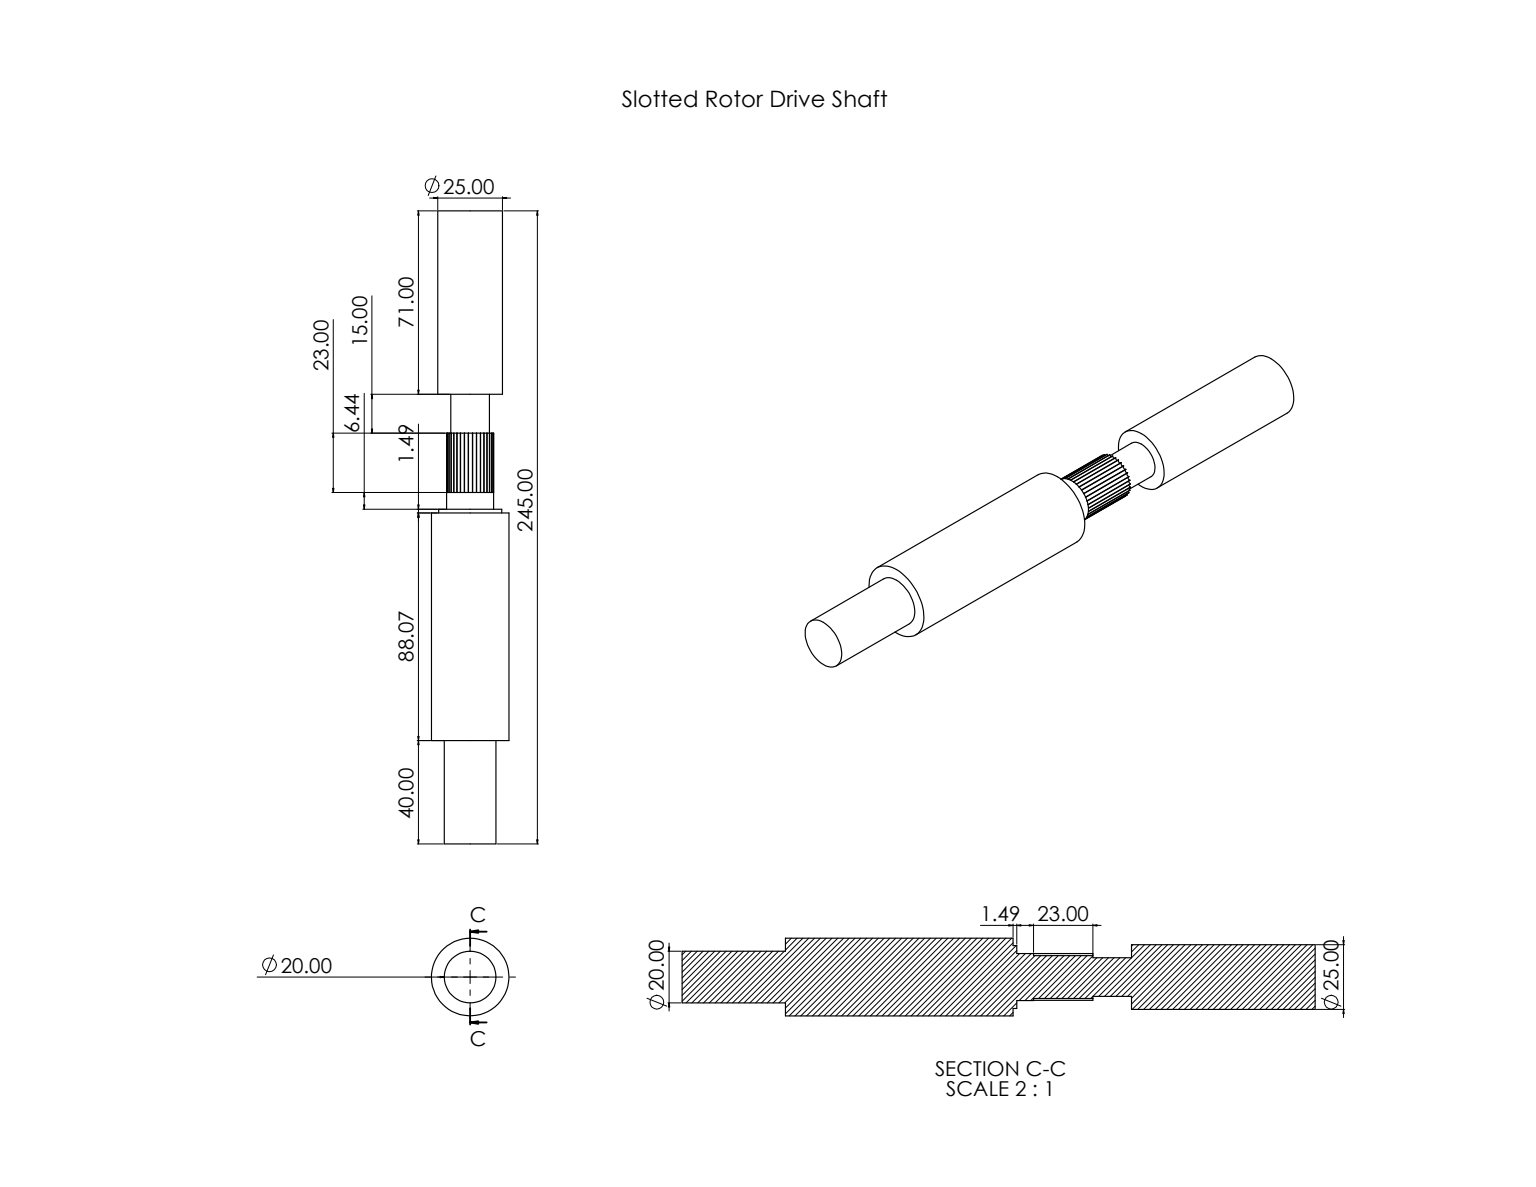
ISO-10303-21;
HEADER;
FILE_DESCRIPTION (('STEP AP214'),
    '1' );
FILE_NAME ('Slotted Rotor Drive Shaft.step',
    '2026-10-18T20:16:25',
    ( '' ),
    ( '' ),
    'SwSTEP 2.0',
    'SolidWorks 2025',
    '' );
FILE_SCHEMA (( 'AUTOMOTIVE_DESIGN' ));
ENDSEC;

DATA;
#10=DIRECTION ( 'NONE',  ( 1.000000000000000000, 0.000000000000000000, 0.000000000000000000 ) ) ;
#12=DIRECTION ( 'NONE',  ( 1.000000000000000000, 0.000000000000000000, 0.000000000000000000 ) ) ;
#34=VERTEX_POINT ( 'NONE', #489 ) ;
#36=DIRECTION ( 'NONE',  ( -0.000000000000000000, -0.000000000000000000, 1.000000000000000000 ) ) ;
#44=LINE ( 'NONE', #17187, #10483 ) ;
#51=CARTESIAN_POINT ( 'NONE',  ( 6.812559277181973627, -5.881244434206257310, 21.50000000000000000 ) ) ;
#57=DIRECTION ( 'NONE',  ( -0.000000000000000000, -0.000000000000000000, 1.000000000000000000 ) ) ;
#88=DIRECTION ( 'NONE',  ( 1.000000000000000000, 0.000000000000000000, 0.000000000000000000 ) ) ;
#89=ORIENTED_EDGE ( 'NONE', *, *, #20188, .F. ) ;
#101=CARTESIAN_POINT ( 'NONE',  ( 0.000000000000000000, 0.000000000000000000, -87.50000000000000000 ) ) ;
#103=ORIENTED_EDGE ( 'NONE', *, *, #23860, .T. ) ;
#107=CYLINDRICAL_SURFACE ( 'NONE', #23715, 10.00000000000003375 ) ;
#120=FACE_OUTER_BOUND ( 'NONE', #29698, .T. ) ;
#128=CARTESIAN_POINT ( 'NONE',  ( 0.000000000000000000, -2.435693370351110282E-15, 21.50000000000000355 ) ) ;
#141=ORIENTED_EDGE ( 'NONE', *, *, #9150, .T. ) ;
#157=ORIENTED_EDGE ( 'NONE', *, *, #6998, .F. ) ;
#163=DIRECTION ( 'NONE',  ( 1.000000000000000000, 0.000000000000000000, -0.000000000000000000 ) ) ;
#167=DIRECTION ( 'NONE',  ( 1.000000000000000000, 0.000000000000000000, 0.000000000000000000 ) ) ;
#168=LINE ( 'NONE', #19198, #17487 ) ;
#181=CARTESIAN_POINT ( 'NONE',  ( 3.993622308618880901, 8.159193615868410632, 21.50000000000000000 ) ) ;
#191=VERTEX_POINT ( 'NONE', #3449 ) ;
#193=CARTESIAN_POINT ( 'NONE',  ( 7.392982946727082449, -5.278755796068694828, -1.500000000000002442 ) ) ;
#222=DIRECTION ( 'NONE',  ( 0.000000000000000000, -1.132880637372608986E-16, 1.000000000000000000 ) ) ;
#233=DIRECTION ( 'NONE',  ( -0.000000000000000000, -0.000000000000000000, 1.000000000000000000 ) ) ;
#246=CARTESIAN_POINT ( 'NONE',  ( -7.856594496258223259, -4.390207617113929039, -1.500000000000002220 ) ) ;
#259=CARTESIAN_POINT ( 'NONE',  ( -8.268028093133393597, -3.763133143576407047, 13.22130136205108819 ) ) ;
#260=DIRECTION ( 'NONE',  ( -0.000000000000000000, 1.132880637372608986E-16, -1.000000000000000000 ) ) ;
#264=ORIENTED_EDGE ( 'NONE', *, *, #13066, .T. ) ;
#275=CIRCLE ( 'NONE', #26685, 10.00000000000003197 ) ;
#280=LINE ( 'NONE', #9800, #11506 ) ;
#299=ORIENTED_EDGE ( 'NONE', *, *, #13066, .F. ) ;
#352=EDGE_LOOP ( 'NONE', ( #24327, #26757, #11753, #27954 ) ) ;
#355=ORIENTED_EDGE ( 'NONE', *, *, #15805, .F. ) ;
#356=CIRCLE ( 'NONE', #4344, 0.7500000000000006661 ) ;
#371=AXIS2_PLACEMENT_3D ( 'NONE', #8358, #11002, #3982 ) ;
#376=EDGE_CURVE ( 'NONE', #10212, #10205, #7649, .T. ) ;
#384=VECTOR ( 'NONE', #1530, 1000.000000000000000 ) ;
#385=EDGE_LOOP ( 'NONE', ( #18527, #8717, #10000, #7620 ) ) ;
#386=VERTEX_POINT ( 'NONE', #5599 ) ;
#394=DIRECTION ( 'NONE',  ( 1.000000000000000000, 0.000000000000000000, -0.000000000000000000 ) ) ;
#396=CYLINDRICAL_SURFACE ( 'NONE', #20666, 0.7500000000000006661 ) ;
#398=ORIENTED_EDGE ( 'NONE', *, *, #13211, .T. ) ;
#411=DIRECTION ( 'NONE',  ( 1.000000000000000000, 0.000000000000000000, 0.000000000000000000 ) ) ;
#419=CARTESIAN_POINT ( 'NONE',  ( -0.6237340761795794331, 8.999114229549594057, -3.621320343559650379 ) ) ;
#426=CIRCLE ( 'NONE', #4407, 0.7500000000000006661 ) ;
#430=CARTESIAN_POINT ( 'NONE',  ( -5.881244434206279514, -6.812559277181949646, -3.621320343559650379 ) ) ;
#449=ADVANCED_FACE ( 'NONE', ( #17752 ), #28148, .F. ) ;
#454=VECTOR ( 'NONE', #3159, 1000.000000000000000 ) ;
#465=DIRECTION ( 'NONE',  ( 0.000000000000000000, -1.132880637372608986E-16, 1.000000000000000000 ) ) ;
#469=CARTESIAN_POINT ( 'NONE',  ( 8.752572334588121450, -2.431858781452763019, 13.22130136205108819 ) ) ;
#472=CARTESIAN_POINT ( 'NONE',  ( 7.856594496258195726, 4.390207617113981442, -3.621320343559650379 ) ) ;
#473=ORIENTED_EDGE ( 'NONE', *, *, #21967, .F. ) ;
#475=PLANE ( 'NONE',  #11721 ) ;
#478=DIRECTION ( 'NONE',  ( 0.000000000000000000, 0.000000000000000000, 1.000000000000000000 ) ) ;
#488=CARTESIAN_POINT ( 'NONE',  ( -2.431858781452794993, -8.752572334588114344, 13.22130136205108641 ) ) ;
#489=CARTESIAN_POINT ( 'NONE',  ( -7.749586724479453181, -2.959227181723774525, 21.50000000000000000 ) ) ;
#495=CIRCLE ( 'NONE', #13480, 0.7500000000000006661 ) ;
#504=CARTESIAN_POINT ( 'NONE',  ( 3.196529495465388226, 8.413215745755008967, 21.50000000000000000 ) ) ;
#507=ORIENTED_EDGE ( 'NONE', *, *, #26727, .T. ) ;
#513=EDGE_LOOP ( 'NONE', ( #8393, #2746, #22053, #19738 ) ) ;
#520=CARTESIAN_POINT ( 'NONE',  ( 3.993622308618881789, 8.159193615868410632, 13.22130136205108997 ) ) ;
#525=DIRECTION ( 'NONE',  ( -0.000000000000000000, -0.000000000000000000, 1.000000000000000000 ) ) ;
#533=PLANE ( 'NONE',  #14075 ) ;
#543=CARTESIAN_POINT ( 'NONE',  ( -3.914781618004754105, -8.197313248159934673, 13.22130136205108641 ) ) ;
#545=CARTESIAN_POINT ( 'NONE',  ( 5.278755796068665518, 7.392982946727100213, 13.22130136205108819 ) ) ;
#549=VERTEX_POINT ( 'NONE', #2245 ) ;
#556=ORIENTED_EDGE ( 'NONE', *, *, #19301, .T. ) ;
#557=DIRECTION ( 'NONE',  ( 0.000000000000000000, -1.132880637372608986E-16, 1.000000000000000000 ) ) ;
#564=DIRECTION ( 'NONE',  ( -0.000000000000000000, 1.132880637372608986E-16, -1.000000000000000000 ) ) ;
#583=DIRECTION ( 'NONE',  ( -0.000000000000000000, -0.000000000000000000, 1.000000000000000000 ) ) ;
#594=CIRCLE ( 'NONE', #15544, 9.084132297865673777 ) ;
#600=PLANE ( 'NONE',  #26319 ) ;
#604=CARTESIAN_POINT ( 'NONE',  ( 0.000000000000000000, -1.324687536737320328E-14, 29.43090101791767665 ) ) ;
#608=CARTESIAN_POINT ( 'NONE',  ( 0.000000000000000000, -2.435693370351110282E-15, 21.50000000000000355 ) ) ;
#610=AXIS2_PLACEMENT_3D ( 'NONE', #14293, #4786, #30528 ) ;
#620=EDGE_CURVE ( 'NONE', #21542, #7918, #19871, .T. ) ;
#630=VECTOR ( 'NONE', #11453, 1000.000000000000000 ) ;
#642=ORIENTED_EDGE ( 'NONE', *, *, #3488, .T. ) ;
#650=CARTESIAN_POINT ( 'NONE',  ( 0.000000000000000000, 12.49999999999999289, -16.50000000000000000 ) ) ;
#651=CARTESIAN_POINT ( 'NONE',  ( 8.499586724479435418, 2.959227181723830036, 21.50000000000000000 ) ) ;
#657=LINE ( 'NONE', #10172, #27987 ) ;
#662=LINE ( 'NONE', #10032, #18671 ) ;
#677=DIRECTION ( 'NONE',  ( 0.000000000000000000, 1.000000000000000000, 0.000000000000000000 ) ) ;
#683=DIRECTION ( 'NONE',  ( 1.000000000000000000, 0.000000000000000000, -0.000000000000000000 ) ) ;
#688=EDGE_LOOP ( 'NONE', ( #7959, #30091, #6151, #14785 ) ) ;
#699=VERTEX_POINT ( 'NONE', #22362 ) ;
#710=CARTESIAN_POINT ( 'NONE',  ( 0.8750451464062524165, 9.041888939645138734, 13.22130136205108997 ) ) ;
#713=CARTESIAN_POINT ( 'NONE',  ( 0.000000000000000000, 0.000000000000000000, -87.50000000000000000 ) ) ;
#726=ORIENTED_EDGE ( 'NONE', *, *, #23506, .T. ) ;
#729=ORIENTED_EDGE ( 'NONE', *, *, #10664, .F. ) ;
#742=CARTESIAN_POINT ( 'NONE',  ( -6.974883619896829146, -5.687793815610328707, 21.50000000000000000 ) ) ;
#743=DIRECTION ( 'NONE',  ( 0.000000000000000000, -1.132880637372608986E-16, 1.000000000000000000 ) ) ;
#753=ORIENTED_EDGE ( 'NONE', *, *, #1735, .F. ) ;
#765=ADVANCED_FACE ( 'NONE', ( #29389 ), #24224, .F. ) ;
#767=DIRECTION ( 'NONE',  ( 0.000000000000000000, 1.132880637372608986E-16, -1.000000000000000000 ) ) ;
#783=CIRCLE ( 'NONE', #24698, 0.7500000000000003331 ) ;
#789=EDGE_CURVE ( 'NONE', #27491, #28009, #15615, .T. ) ;
#795=ADVANCED_FACE ( 'NONE', ( #1471 ), #25006, .F. ) ;
#796=ORIENTED_EDGE ( 'NONE', *, *, #17613, .F. ) ;
#798=DIRECTION ( 'NONE',  ( -0.000000000000000000, 1.132880637372608986E-16, -1.000000000000000000 ) ) ;
#804=FACE_OUTER_BOUND ( 'NONE', #18026, .T. ) ;
#808=DIRECTION ( 'NONE',  ( -0.000000000000000000, 1.132880637372608986E-16, -1.000000000000000000 ) ) ;
#823=EDGE_CURVE ( 'NONE', #12314, #11064, #25600, .T. ) ;
#831=CIRCLE ( 'NONE', #11309, 7.500000000000007105 ) ;
#853=ORIENTED_EDGE ( 'NONE', *, *, #25955, .F. ) ;
#858=ORIENTED_EDGE ( 'NONE', *, *, #7497, .F. ) ;
#868=EDGE_CURVE ( 'NONE', #29154, #3530, #21387, .T. ) ;
#877=AXIS2_PLACEMENT_3D ( 'NONE', #2661, #478, #28713 ) ;
#880=CARTESIAN_POINT ( 'NONE',  ( -8.268028093133395373, -3.763133143576407935, 21.50000000000000000 ) ) ;
#890=CARTESIAN_POINT ( 'NONE',  ( 8.884323311075775109, 1.438332125858202692, -1.500000000000001776 ) ) ;
#897=VERTEX_POINT ( 'NONE', #21221 ) ;
#901=CIRCLE ( 'NONE', #26810, 0.7499999999999997780 ) ;
#903=ORIENTED_EDGE ( 'NONE', *, *, #17740, .F. ) ;
#919=DIRECTION ( 'NONE',  ( 0.000000000000000000, 1.000000000000000000, 0.000000000000000000 ) ) ;
#928=DIRECTION ( 'NONE',  ( 0.000000000000000000, 1.000000000000000000, 0.000000000000000000 ) ) ;
#931=ORIENTED_EDGE ( 'NONE', *, *, #11263, .T. ) ;
#939=CIRCLE ( 'NONE', #18392, 15.00000000000003375 ) ;
#949=CIRCLE ( 'NONE', #4929, 0.7500000000000003331 ) ;
#1004=DIRECTION ( 'NONE',  ( 0.000000000000000000, 0.000000000000000000, 1.000000000000000000 ) ) ;
#1011=ORIENTED_EDGE ( 'NONE', *, *, #6998, .T. ) ;
#1021=ORIENTED_EDGE ( 'NONE', *, *, #620, .T. ) ;
#1022=CARTESIAN_POINT ( 'NONE',  ( 5.069257791428380955, -7.538175180318438251, -1.500000000000002665 ) ) ;
#1023=EDGE_CURVE ( 'NONE', #4256, #10933, #14676, .T. ) ;
#1032=CARTESIAN_POINT ( 'NONE',  ( -2.185336383880142730, 8.817355867515834333, -1.500000000000000666 ) ) ;
#1033=VERTEX_POINT ( 'NONE', #5324 ) ;
#1056=DIRECTION ( 'NONE',  ( 1.000000000000000000, 0.000000000000000000, -0.000000000000000000 ) ) ;
#1058=EDGE_LOOP ( 'NONE', ( #9791, #10369, #20213, #24260 ) ) ;
#1063=AXIS2_PLACEMENT_3D ( 'NONE', #16979, #17133, #5749 ) ;
#1065=ORIENTED_EDGE ( 'NONE', *, *, #20188, .T. ) ;
#1082=ORIENTED_EDGE ( 'NONE', *, *, #23253, .T. ) ;
#1084=CARTESIAN_POINT ( 'NONE',  ( -8.728722367416567707, 2.516121109503271835, -1.500000000000001554 ) ) ;
#1104=CIRCLE ( 'NONE', #15024, 9.084132297865673777 ) ;
#1124=DIRECTION ( 'NONE',  ( -0.000000000000000000, 1.132880637372608986E-16, -1.000000000000000000 ) ) ;
#1159=ADVANCED_FACE ( 'NONE', ( #13126 ), #5948, .F. ) ;
#1163=CIRCLE ( 'NONE', #17097, 9.084132297865673777 ) ;
#1166=DIRECTION ( 'NONE',  ( 1.000000000000000000, 0.000000000000000000, 0.000000000000000000 ) ) ;
#1183=VECTOR ( 'NONE', #12787, 1000.000000000000000 ) ;
#1192=DIRECTION ( 'NONE',  ( -0.000000000000000000, 1.132880637372608986E-16, -1.000000000000000000 ) ) ;
#1193=DIRECTION ( 'NONE',  ( 0.000000000000000000, 1.000000000000000000, 0.000000000000000000 ) ) ;
#1194=DIRECTION ( 'NONE',  ( -0.000000000000000000, 1.132880637372608986E-16, -1.000000000000000000 ) ) ;
#1195=CARTESIAN_POINT ( 'NONE',  ( -1.687027447297492211, -8.840471615930066918, -3.621320343559650379 ) ) ;
#1196=DIRECTION ( 'NONE',  ( 1.000000000000000000, 0.000000000000000000, 0.000000000000000000 ) ) ;
#1197=ORIENTED_EDGE ( 'NONE', *, *, #17988, .F. ) ;
#1209=CARTESIAN_POINT ( 'NONE',  ( -8.795879380940579750, -2.270234684139648795, 13.22130136205108819 ) ) ;
#1214=ADVANCED_FACE ( 'NONE', ( #7629 ), #12629, .T. ) ;
#1220=CARTESIAN_POINT ( 'NONE',  ( -5.881244434206279514, -6.812559277181949646, -1.500000000000002665 ) ) ;
#1226=AXIS2_PLACEMENT_3D ( 'NONE', #23821, #14627, #4503 ) ;
#1228=ADVANCED_FACE ( 'NONE', ( #29312 ), #600, .F. ) ;
#1232=EDGE_CURVE ( 'NONE', #6203, #13370, #19780, .T. ) ;
#1237=ORIENTED_EDGE ( 'NONE', *, *, #20788, .T. ) ;
#1247=DIRECTION ( 'NONE',  ( 0.000000000000000000, 1.132880637372608986E-16, -1.000000000000000000 ) ) ;
#1261=ORIENTED_EDGE ( 'NONE', *, *, #10902, .T. ) ;
#1271=ORIENTED_EDGE ( 'NONE', *, *, #17391, .F. ) ;
#1289=CARTESIAN_POINT ( 'NONE',  ( 8.840471615930072247, -1.687027447297460236, 21.50000000000000000 ) ) ;
#1294=VECTOR ( 'NONE', #26040, 1000.000000000000000 ) ;
#1306=CARTESIAN_POINT ( 'NONE',  ( -0.8750451464063155882, -9.041888939645136958, 13.22130136205108641 ) ) ;
#1314=VERTEX_POINT ( 'NONE', #19950 ) ;
#1330=CIRCLE ( 'NONE', #18761, 9.084132297865673777 ) ;
#1331=VECTOR ( 'NONE', #23455, 1000.000000000000000 ) ;
#1333=CIRCLE ( 'NONE', #4815, 0.7500000000000006661 ) ;
#1337=DIRECTION ( 'NONE',  ( 0.000000000000000000, -1.132880637372608986E-16, 1.000000000000000000 ) ) ;
#1344=CARTESIAN_POINT ( 'NONE',  ( 0.000000000000000000, 8.021365865836055733E-32, -87.50000000000000000 ) ) ;
#1375=VERTEX_POINT ( 'NONE', #14486 ) ;
#1380=ORIENTED_EDGE ( 'NONE', *, *, #22384, .F. ) ;
#1404=CYLINDRICAL_SURFACE ( 'NONE', #3158, 0.7500000000000007772 ) ;
#1409=DIRECTION ( 'NONE',  ( 0.000000000000000000, 1.132880637372608986E-16, -1.000000000000000000 ) ) ;
#1410=DIRECTION ( 'NONE',  ( -0.000000000000000000, -0.000000000000000000, 1.000000000000000000 ) ) ;
#1420=CARTESIAN_POINT ( 'NONE',  ( -2.270234684139619485, 8.795879380940585079, 21.50000000000000000 ) ) ;
#1426=ORIENTED_EDGE ( 'NONE', *, *, #17426, .T. ) ;
#1436=CYLINDRICAL_SURFACE ( 'NONE', #9348, 0.7499999999999997780 ) ;
#1438=ORIENTED_EDGE ( 'NONE', *, *, #7875, .T. ) ;
#1447=CARTESIAN_POINT ( 'NONE',  ( 0.000000000000000000, -2.435693370351110282E-15, 21.50000000000000355 ) ) ;
#1451=ADVANCED_FACE ( 'NONE', ( #8871 ), #6375, .F. ) ;
#1454=EDGE_LOOP ( 'NONE', ( #21314, #26779, #24672, #6275 ) ) ;
#1456=CARTESIAN_POINT ( 'NONE',  ( -7.488956955540436056, -5.141690706682852330, -1.500000000000002442 ) ) ;
#1458=VERTEX_POINT ( 'NONE', #22735 ) ;
#1471=FACE_OUTER_BOUND ( 'NONE', #1058, .T. ) ;
#1472=ORIENTED_EDGE ( 'NONE', *, *, #24991, .T. ) ;
#1492=ORIENTED_EDGE ( 'NONE', *, *, #28292, .F. ) ;
#1493=CIRCLE ( 'NONE', #9942, 0.7500000000000006661 ) ;
#1496=ORIENTED_EDGE ( 'NONE', *, *, #13412, .F. ) ;
#1500=DIRECTION ( 'NONE',  ( 0.000000000000000000, -1.132880637372608986E-16, 1.000000000000000000 ) ) ;
#1508=FACE_OUTER_BOUND ( 'NONE', #28742, .T. ) ;
#1509=CARTESIAN_POINT ( 'NONE',  ( 1.687027447297431371, 8.840471615930075799, -3.621320343559650379 ) ) ;
#1517=DIRECTION ( 'NONE',  ( 0.000000000000000000, -1.132880637372608986E-16, 1.000000000000000000 ) ) ;
#1521=EDGE_CURVE ( 'NONE', #28904, #8444, #426, .T. ) ;
#1522=ORIENTED_EDGE ( 'NONE', *, *, #24101, .F. ) ;
#1530=DIRECTION ( 'NONE',  ( -0.000000000000000000, 1.132880637372608986E-16, -1.000000000000000000 ) ) ;
#1533=AXIS2_PLACEMENT_3D ( 'NONE', #5893, #583, #10420 ) ;
#1543=ORIENTED_EDGE ( 'NONE', *, *, #27881, .T. ) ;
#1549=EDGE_CURVE ( 'NONE', #19074, #19937, #8411, .T. ) ;
#1555=CIRCLE ( 'NONE', #2046, 0.7499999999999997780 ) ;
#1559=VERTEX_POINT ( 'NONE', #23806 ) ;
#1560=EDGE_CURVE ( 'NONE', #2431, #1375, #11898, .T. ) ;
#1565=DIRECTION ( 'NONE',  ( 1.000000000000000000, 0.000000000000000000, 0.000000000000000000 ) ) ;
#1566=ORIENTED_EDGE ( 'NONE', *, *, #24828, .F. ) ;
#1578=VECTOR ( 'NONE', #3789, 1000.000000000000000 ) ;
#1584=DIRECTION ( 'NONE',  ( 0.000000000000000000, -1.132880637372608986E-16, 1.000000000000000000 ) ) ;
#1587=ORIENTED_EDGE ( 'NONE', *, *, #7500, .T. ) ;
#1593=CARTESIAN_POINT ( 'NONE',  ( 8.884323311075775109, 1.438332125858202692, 21.50000000000000000 ) ) ;
#1601=EDGE_CURVE ( 'NONE', #9461, #16202, #8925, .T. ) ;
#1623=EDGE_CURVE ( 'NONE', #26855, #21196, #9024, .T. ) ;
#1624=AXIS2_PLACEMENT_3D ( 'NONE', #8813, #25347, #23302 ) ;
#1638=EDGE_LOOP ( 'NONE', ( #27726, #29523, #9939 ) ) ;
#1644=ORIENTED_EDGE ( 'NONE', *, *, #2360, .T. ) ;
#1647=ORIENTED_EDGE ( 'NONE', *, *, #1560, .F. ) ;
#1657=CARTESIAN_POINT ( 'NONE',  ( -8.840471615930058036, 1.687027447297517080, -3.621320343559650379 ) ) ;
#1661=VERTEX_POINT ( 'NONE', #25551 ) ;
#1662=VERTEX_POINT ( 'NONE', #4176 ) ;
#1665=VERTEX_POINT ( 'NONE', #25860 ) ;
#1673=DIRECTION ( 'NONE',  ( 0.000000000000000000, -1.132880637372608986E-16, 1.000000000000000000 ) ) ;
#1679=DIRECTION ( 'NONE',  ( -0.000000000000000000, -0.000000000000000000, 1.000000000000000000 ) ) ;
#1692=VERTEX_POINT ( 'NONE', #13704 ) ;
#1694=CARTESIAN_POINT ( 'NONE',  ( -2.431858781452794993, -8.752572334588114344, 21.50000000000000000 ) ) ;
#1699=DIRECTION ( 'NONE',  ( 1.000000000000000000, 0.000000000000000000, -0.000000000000000000 ) ) ;
#1700=ORIENTED_EDGE ( 'NONE', *, *, #22914, .F. ) ;
#1703=ORIENTED_EDGE ( 'NONE', *, *, #13989, .F. ) ;
#1706=ORIENTED_EDGE ( 'NONE', *, *, #15656, .T. ) ;
#1717=CARTESIAN_POINT ( 'NONE',  ( 1.438332125858173605, -8.884323311075778662, -3.621320343559650379 ) ) ;
#1720=ADVANCED_FACE ( 'NONE', ( #21149 ), #30669, .F. ) ;
#1723=DIRECTION ( 'NONE',  ( -0.000000000000000000, -0.000000000000000000, 1.000000000000000000 ) ) ;
#1735=EDGE_CURVE ( 'NONE', #4121, #4711, #16798, .T. ) ;
#1742=CYLINDRICAL_SURFACE ( 'NONE', #11330, 0.7500000000000007772 ) ;
#1744=FACE_OUTER_BOUND ( 'NONE', #18324, .T. ) ;
#1746=DIRECTION ( 'NONE',  ( 1.000000000000000000, 0.000000000000000000, 0.000000000000000000 ) ) ;
#1762=ADVANCED_FACE ( 'NONE', ( #9938, #26790 ), #19141, .T. ) ;
#1773=AXIS2_PLACEMENT_3D ( 'NONE', #23243, #11876, #18449 ) ;
#1790=EDGE_CURVE ( 'NONE', #20003, #11001, #16858, .T. ) ;
#1808=DIRECTION ( 'NONE',  ( -0.000000000000000000, 1.132880637372608986E-16, -1.000000000000000000 ) ) ;
#1813=AXIS2_PLACEMENT_3D ( 'NONE', #19674, #10322, #8151 ) ;
#1825=EDGE_CURVE ( 'NONE', #30853, #15826, #19864, .T. ) ;
#1830=CARTESIAN_POINT ( 'NONE',  ( 0.000000000000000000, 1.699320956058915452E-16, -1.500000000000001776 ) ) ;
#1832=AXIS2_PLACEMENT_3D ( 'NONE', #30006, #11583, #28276 ) ;
#1840=CYLINDRICAL_SURFACE ( 'NONE', #3816, 12.50000000000000000 ) ;
#1859=EDGE_CURVE ( 'NONE', #11064, #12314, #939, .T. ) ;
#1860=CARTESIAN_POINT ( 'NONE',  ( 0.000000000000000000, 1.699320956058915452E-16, -1.500000000000001776 ) ) ;
#1903=VERTEX_POINT ( 'NONE', #27087 ) ;
#1909=EDGE_CURVE ( 'NONE', #26525, #23603, #11392, .T. ) ;
#1916=ORIENTED_EDGE ( 'NONE', *, *, #18398, .F. ) ;
#1922=ORIENTED_EDGE ( 'NONE', *, *, #25410, .F. ) ;
#1925=ADVANCED_FACE ( 'NONE', ( #15845 ), #27406, .F. ) ;
#1927=EDGE_CURVE ( 'NONE', #21957, #15560, #26866, .T. ) ;
#1928=CARTESIAN_POINT ( 'NONE',  ( 0.8762659238204211221, 8.999114229549594057, -3.621320343559650379 ) ) ;
#1939=CIRCLE ( 'NONE', #11900, 9.084132297865673777 ) ;
#1940=DIRECTION ( 'NONE',  ( 0.000000000000000000, 0.000000000000000000, 1.000000000000000000 ) ) ;
#1941=EDGE_LOOP ( 'NONE', ( #5294, #26095 ) ) ;
#1943=DIRECTION ( 'NONE',  ( 0.000000000000000000, -1.132880637372608986E-16, 1.000000000000000000 ) ) ;
#1944=ADVANCED_FACE ( 'NONE', ( #20059 ), #29898, .F. ) ;
#1950=ADVANCED_FACE ( 'NONE', ( #20519, #3379 ), #29581, .T. ) ;
#1952=FACE_OUTER_BOUND ( 'NONE', #6640, .T. ) ;
#1968=VERTEX_POINT ( 'NONE', #11772 ) ;
#1983=EDGE_CURVE ( 'NONE', #12192, #18134, #25856, .T. ) ;
#1990=DIRECTION ( 'NONE',  ( 0.000000000000000000, 0.000000000000000000, 1.000000000000000000 ) ) ;
#1996=ORIENTED_EDGE ( 'NONE', *, *, #20841, .T. ) ;
#1999=ADVANCED_FACE ( 'NONE', ( #11327 ), #14249, .F. ) ;
#2025=VECTOR ( 'NONE', #25260, 1000.000000000000000 ) ;
#2031=EDGE_CURVE ( 'NONE', #29358, #9984, #26365, .T. ) ;
#2036=CARTESIAN_POINT ( 'NONE',  ( -1.438332125858111432, 8.884323311075791096, -3.621320343559650379 ) ) ;
#2044=EDGE_LOOP ( 'NONE', ( #2535, #19126, #18814, #3222 ) ) ;
#2046=AXIS2_PLACEMENT_3D ( 'NONE', #10083, #19596, #29117 ) ;
#2051=CARTESIAN_POINT ( 'NONE',  ( 2.185336383880203570, -8.817355867515820123, -1.500000000000002887 ) ) ;
#2052=DIRECTION ( 'NONE',  ( 0.000000000000000000, 0.000000000000000000, 1.000000000000000000 ) ) ;
#2054=DIRECTION ( 'NONE',  ( 0.000000000000000000, 0.000000000000000000, 1.000000000000000000 ) ) ;
#2061=EDGE_LOOP ( 'NONE', ( #19925, #1644, #18712, #22600 ) ) ;
#2068=CARTESIAN_POINT ( 'NONE',  ( 6.812559277181973627, -5.881244434206257310, -1.500000000000002220 ) ) ;
#2095=DIRECTION ( 'NONE',  ( 1.000000000000000000, 0.000000000000000000, -0.000000000000000000 ) ) ;
#2096=EDGE_CURVE ( 'NONE', #11840, #29091, #8440, .T. ) ;
#2098=LINE ( 'NONE', #8984, #28287 ) ;
#2107=ORIENTED_EDGE ( 'NONE', *, *, #3911, .F. ) ;
#2118=VERTEX_POINT ( 'NONE', #17813 ) ;
#2124=DIRECTION ( 'NONE',  ( 0.000000000000000000, 0.000000000000000000, 1.000000000000000000 ) ) ;
#2128=CARTESIAN_POINT ( 'NONE',  ( 8.413215745754998309, -3.196529495465417980, -3.621320343559650379 ) ) ;
#2147=ORIENTED_EDGE ( 'NONE', *, *, #15449, .T. ) ;
#2148=ORIENTED_EDGE ( 'NONE', *, *, #10232, .T. ) ;
#2166=AXIS2_PLACEMENT_3D ( 'NONE', #17378, #7866, #26899 ) ;
#2196=ORIENTED_EDGE ( 'NONE', *, *, #15690, .F. ) ;
#2212=ORIENTED_EDGE ( 'NONE', *, *, #23274, .T. ) ;
#2229=DIRECTION ( 'NONE',  ( 1.000000000000000000, 0.000000000000000000, 0.000000000000000000 ) ) ;
#2239=DIRECTION ( 'NONE',  ( 1.000000000000000000, 0.000000000000000000, 0.000000000000000000 ) ) ;
#2245=CARTESIAN_POINT ( 'NONE',  ( 1.224646799147357201E-15, -10.00000000000005329, 117.5000000000000000 ) ) ;
#2257=CYLINDRICAL_SURFACE ( 'NONE', #24911, 0.7500000000000006661 ) ;
#2272=VERTEX_POINT ( 'NONE', #15535 ) ;
#2288=CARTESIAN_POINT ( 'NONE',  ( -7.730328572437709767, 4.608906612435681005, 21.50000000000000000 ) ) ;
#2294=AXIS2_PLACEMENT_3D ( 'NONE', #25091, #27442, #6218 ) ;
#2301=EDGE_CURVE ( 'NONE', #19148, #6231, #13523, .T. ) ;
#2303=ORIENTED_EDGE ( 'NONE', *, *, #20028, .T. ) ;
#2335=DIRECTION ( 'NONE',  ( 0.000000000000000000, -1.132880637372608986E-16, 1.000000000000000000 ) ) ;
#2336=DIRECTION ( 'NONE',  ( 0.000000000000000000, 1.000000000000000000, 1.156482317317869999E-16 ) ) ;
#2345=DIRECTION ( 'NONE',  ( 0.000000000000000000, 0.000000000000000000, 1.000000000000000000 ) ) ;
#2351=AXIS2_PLACEMENT_3D ( 'NONE', #25921, #6892, #16406 ) ;
#2352=DIRECTION ( 'NONE',  ( 0.000000000000000000, 0.000000000000000000, 1.000000000000000000 ) ) ;
#2360=EDGE_CURVE ( 'NONE', #14759, #11459, #10203, .T. ) ;
#2363=CARTESIAN_POINT ( 'NONE',  ( 0.9621688436939446198, 9.033033306777459970, -1.500000000000000666 ) ) ;
#2364=AXIS2_PLACEMENT_3D ( 'NONE', #4195, #30096, #18246 ) ;
#2367=DIRECTION ( 'NONE',  ( 6.216092455583553496E-15, 1.000000000000000000, 0.000000000000000000 ) ) ;
#2374=PLANE ( 'NONE',  #15534 ) ;
#2390=DIRECTION ( 'NONE',  ( 1.000000000000000000, 0.000000000000000000, -0.000000000000000000 ) ) ;
#2407=VECTOR ( 'NONE', #19625, 1000.000000000000000 ) ;
#2416=CARTESIAN_POINT ( 'NONE',  ( 9.033033306777456417, -0.9621688436939739297, 13.22130136205108819 ) ) ;
#2431=VERTEX_POINT ( 'NONE', #20025 ) ;
#2437=DIRECTION ( 'NONE',  ( 0.000000000000000000, 1.132880637372608986E-16, -1.000000000000000000 ) ) ;
#2455=DIRECTION ( 'NONE',  ( 0.000000000000000000, 1.000000000000000000, 0.000000000000000000 ) ) ;
#2461=AXIS2_PLACEMENT_3D ( 'NONE', #6539, #11067, #13262 ) ;
#2464=ORIENTED_EDGE ( 'NONE', *, *, #29382, .F. ) ;
#2481=ORIENTED_EDGE ( 'NONE', *, *, #12580, .F. ) ;
#2494=ORIENTED_EDGE ( 'NONE', *, *, #376, .T. ) ;
#2495=VERTEX_POINT ( 'NONE', #3654 ) ;
#2500=DIRECTION ( 'NONE',  ( 0.000000000000000000, -1.132880637372608986E-16, 1.000000000000000000 ) ) ;
#2512=AXIS2_PLACEMENT_3D ( 'NONE', #27208, #29400, #8513 ) ;
#2514=ORIENTED_EDGE ( 'NONE', *, *, #24608, .F. ) ;
#2519=CYLINDRICAL_SURFACE ( 'NONE', #12031, 0.7499999999999997780 ) ;
#2522=CARTESIAN_POINT ( 'NONE',  ( 0.000000000000000000, -2.435693370351110282E-15, 21.50000000000000355 ) ) ;
#2529=EDGE_CURVE ( 'NONE', #20718, #8541, #24039, .T. ) ;
#2535=ORIENTED_EDGE ( 'NONE', *, *, #24634, .F. ) ;
#2539=EDGE_CURVE ( 'NONE', #6919, #11684, #5300, .T. ) ;
#2547=VERTEX_POINT ( 'NONE', #19378 ) ;
#2587=VERTEX_POINT ( 'NONE', #26556 ) ;
#2597=CARTESIAN_POINT ( 'NONE',  ( 0.000000000000000000, 1.699320956058915452E-16, -1.500000000000001776 ) ) ;
#2598=CARTESIAN_POINT ( 'NONE',  ( 8.159193615868399974, -3.993622308618911099, 21.50000000000000000 ) ) ;
#2602=EDGE_CURVE ( 'NONE', #1033, #2495, #21218, .T. ) ;
#2628=ADVANCED_FACE ( 'NONE', ( #5184 ), #7209, .F. ) ;
#2632=CYLINDRICAL_SURFACE ( 'NONE', #30688, 0.7500000000000006661 ) ;
#2639=AXIS2_PLACEMENT_3D ( 'NONE', #24872, #13169, #18314 ) ;
#2649=CARTESIAN_POINT ( 'NONE',  ( -6.543385983536391670, -6.301234758012574488, 21.50000000000000000 ) ) ;
#2653=ORIENTED_EDGE ( 'NONE', *, *, #27879, .F. ) ;
#2659=CARTESIAN_POINT ( 'NONE',  ( -9.041888939645129852, 0.8750451464063455642, 21.50000000000000000 ) ) ;
#2661=CARTESIAN_POINT ( 'NONE',  ( -1.438332125858111432, 8.884323311075791096, 21.50000000000000000 ) ) ;
#2662=AXIS2_PLACEMENT_3D ( 'NONE', #21189, #28233, #9363 ) ;
#2663=ORIENTED_EDGE ( 'NONE', *, *, #13799, .F. ) ;
#2665=AXIS2_PLACEMENT_3D ( 'NONE', #19796, #19492, #7643 ) ;
#2666=CARTESIAN_POINT ( 'NONE',  ( -0.8762659238204844048, -8.999114229549588728, -3.621320343559650379 ) ) ;
#2671=DIRECTION ( 'NONE',  ( 1.000000000000000000, 0.000000000000000000, 0.000000000000000000 ) ) ;
#2678=EDGE_CURVE ( 'NONE', #1559, #5756, #14256, .T. ) ;
#2687=CIRCLE ( 'NONE', #23024, 0.7499999999999997780 ) ;
#2691=CARTESIAN_POINT ( 'NONE',  ( 8.840471615930072247, -1.687027447297460236, -1.500000000000001776 ) ) ;
#2706=EDGE_CURVE ( 'NONE', #19691, #14477, #14997, .T. ) ;
#2718=ADVANCED_FACE ( 'NONE', ( #3155 ), #29514, .F. ) ;
#2726=CYLINDRICAL_SURFACE ( 'NONE', #25269, 0.7500000000000006661 ) ;
#2737=CIRCLE ( 'NONE', #21140, 9.084132297865673777 ) ;
#2746=ORIENTED_EDGE ( 'NONE', *, *, #29772, .T. ) ;
#2750=EDGE_CURVE ( 'NONE', #28599, #15594, #13606, .T. ) ;
#2760=FACE_OUTER_BOUND ( 'NONE', #14871, .T. ) ;
#2764=CARTESIAN_POINT ( 'NONE',  ( -9.041888939645131629, 0.8750451464063454532, -1.500000000000001776 ) ) ;
#2771=ORIENTED_EDGE ( 'NONE', *, *, #19128, .T. ) ;
#2785=EDGE_LOOP ( 'NONE', ( #7545, #15397, #16742, #26570, #2825, #18043, #18666, #5261, #18183, #2212, #30049, #12946, #28144, #12594, #5941, #25114, #642, #26416, #14017, #22966, #13161, #25380, #8556, #5844, #30157, #15989, #2771, #29412, #264, #5315, #3402, #11302, #8012, #16424, #13465, #17720, #23164, #4953, #14913, #11508, #1543, #13383, #11078, #21358, #19015, #1706, #9184, #29602, #23286, #3211, #26176, #13722, #29710, #23357, #17012, #7602, #1472, #9361, #9914, #29202, #28662, #2303, #8298, #4741, #19269, #28525, #18303, #16905, #28327, #15076, #15954, #1237, #3116, #19448, #25267, #27921, #15400, #13152, #23373, #15189, #4461, #15161, #21555, #3551, #12990, #5832, #27207, #10991, #30658, #6470, #21210, #24368, #13252 ) ) ;
#2801=ORIENTED_EDGE ( 'NONE', *, *, #7673, .F. ) ;
#2807=AXIS2_PLACEMENT_3D ( 'NONE', #3105, #743, #29145 ) ;
#2809=DIRECTION ( 'NONE',  ( -0.000000000000000000, -0.000000000000000000, 1.000000000000000000 ) ) ;
#2811=MANIFOLD_SOLID_BREP ( 'Cut-Extrude25', #25765 ) ;
#2819=ORIENTED_EDGE ( 'NONE', *, *, #4616, .T. ) ;
#2825=ORIENTED_EDGE ( 'NONE', *, *, #4464, .T. ) ;
#2845=DIRECTION ( 'NONE',  ( 0.000000000000000000, -1.132880637372608986E-16, 1.000000000000000000 ) ) ;
#2851=DIRECTION ( 'NONE',  ( 0.000000000000000000, 0.000000000000000000, 1.000000000000000000 ) ) ;
#2865=CARTESIAN_POINT ( 'NONE',  ( 0.000000000000000000, -8.043452525345523162E-15, -16.50000000000000000 ) ) ;
#2878=CARTESIAN_POINT ( 'NONE',  ( -5.069257791428325888, 7.538175180318473778, 21.50000000000000000 ) ) ;
#2880=LINE ( 'NONE', #12404, #29231 ) ;
#2897=SHAPE_DEFINITION_REPRESENTATION ( #11653, #23229 ) ;
#2905=CARTESIAN_POINT ( 'NONE',  ( -8.752572334588103686, 2.431858781452820306, 21.50000000000000000 ) ) ;
#2920=CARTESIAN_POINT ( 'NONE',  ( -6.301234758012549619, 6.543385983536412098, 21.50000000000000000 ) ) ;
#2932=ORIENTED_EDGE ( 'NONE', *, *, #28839, .T. ) ;
#2934=ADVANCED_FACE ( 'NONE', ( #30661 ), #11361, .T. ) ;
#2944=ORIENTED_EDGE ( 'NONE', *, *, #19013, .T. ) ;
#2948=ORIENTED_EDGE ( 'NONE', *, *, #14661, .F. ) ;
#2950=ORIENTED_EDGE ( 'NONE', *, *, #17613, .T. ) ;
#2984=DIRECTION ( 'NONE',  ( 1.000000000000000000, 0.000000000000000000, 0.000000000000000000 ) ) ;
#2989=CARTESIAN_POINT ( 'NONE',  ( -8.840471615930058036, 1.687027447297517080, -1.500000000000001776 ) ) ;
#2997=DIRECTION ( 'NONE',  ( 0.000000000000000000, 0.000000000000000000, 1.000000000000000000 ) ) ;
#2998=AXIS2_PLACEMENT_3D ( 'NONE', #26524, #28710, #7187 ) ;
#3025=CARTESIAN_POINT ( 'NONE',  ( -3.640207617113898841, 7.856594496258241023, -3.621320343559650379 ) ) ;
#3039=FACE_OUTER_BOUND ( 'NONE', #2044, .T. ) ;
#3066=DIRECTION ( 'NONE',  ( -1.156482317317871725E-15, 1.000000000000000000, 0.000000000000000000 ) ) ;
#3070=CARTESIAN_POINT ( 'NONE',  ( 0.000000000000000000, 12.49999999999999289, -16.50000000000000000 ) ) ;
#3072=AXIS2_PLACEMENT_3D ( 'NONE', #8414, #30384, #20407 ) ;
#3074=CARTESIAN_POINT ( 'NONE',  ( 6.364020599487797192, -6.482337650448430466, 21.50000000000000000 ) ) ;
#3083=CIRCLE ( 'NONE', #25993, 9.084132297865673777 ) ;
#3105=CARTESIAN_POINT ( 'NONE',  ( -4.608906612435655248, -7.730328572437724866, -1.500000000000002665 ) ) ;
#3116=ORIENTED_EDGE ( 'NONE', *, *, #1601, .T. ) ;
#3131=EDGE_CURVE ( 'NONE', #25497, #6824, #26753, .T. ) ;
#3138=AXIS2_PLACEMENT_3D ( 'NONE', #27047, #24858, #15169 ) ;
#3150=ORIENTED_EDGE ( 'NONE', *, *, #24456, .F. ) ;
#3155=FACE_OUTER_BOUND ( 'NONE', #15975, .T. ) ;
#3157=CARTESIAN_POINT ( 'NONE',  ( -0.9621688436940066813, -9.033033306777454641, 13.22130136205108641 ) ) ;
#3158=AXIS2_PLACEMENT_3D ( 'NONE', #18234, #10916, #20419 ) ;
#3159=DIRECTION ( 'NONE',  ( 0.000000000000000000, -1.132880637372608986E-16, 1.000000000000000000 ) ) ;
#3162=AXIS2_PLACEMENT_3D ( 'NONE', #22289, #1247, #22905 ) ;
#3179=VERTEX_POINT ( 'NONE', #29427 ) ;
#3181=CARTESIAN_POINT ( 'NONE',  ( 2.431858781452735485, 8.752572334588128555, -1.500000000000000666 ) ) ;
#3188=PLANE ( 'NONE',  #23740 ) ;
#3207=ORIENTED_EDGE ( 'NONE', *, *, #28683, .T. ) ;
#3208=DIRECTION ( 'NONE',  ( 0.000000000000000000, 1.000000000000000000, 0.000000000000000000 ) ) ;
#3211=ORIENTED_EDGE ( 'NONE', *, *, #22111, .T. ) ;
#3222=ORIENTED_EDGE ( 'NONE', *, *, #6966, .T. ) ;
#3236=DIRECTION ( 'NONE',  ( 0.000000000000000000, -1.132880637372608986E-16, 1.000000000000000000 ) ) ;
#3245=DIRECTION ( 'NONE',  ( 0.000000000000000000, 0.000000000000000000, 1.000000000000000000 ) ) ;
#3254=VERTEX_POINT ( 'NONE', #11614 ) ;
#3269=AXIS2_PLACEMENT_3D ( 'NONE', #6130, #8777, #6450 ) ;
#3278=DIRECTION ( 'NONE',  ( 1.000000000000000000, 0.000000000000000000, 0.000000000000000000 ) ) ;
#3279=ADVANCED_FACE ( 'NONE', ( #1952 ), #27998, .F. ) ;
#3297=LINE ( 'NONE', #22471, #18767 ) ;
#3305=CYLINDRICAL_SURFACE ( 'NONE', #20358, 0.7500000000000006661 ) ;
#3309=VECTOR ( 'NONE', #19863, 1000.000000000000000 ) ;
#3314=ORIENTED_EDGE ( 'NONE', *, *, #20782, .F. ) ;
#3319=ORIENTED_EDGE ( 'NONE', *, *, #16402, .T. ) ;
#3341=CARTESIAN_POINT ( 'NONE',  ( -8.840471615930058036, 1.687027447297517080, 21.50000000000000000 ) ) ;
#3361=DIRECTION ( 'NONE',  ( -0.000000000000000000, -0.000000000000000000, 1.000000000000000000 ) ) ;
#3374=AXIS2_PLACEMENT_3D ( 'NONE', #25137, #13303, #5658 ) ;
#3375=CIRCLE ( 'NONE', #20798, 0.7500000000000006661 ) ;
#3379=FACE_BOUND ( 'NONE', #5857, .T. ) ;
#3401=CARTESIAN_POINT ( 'NONE',  ( 0.000000000000000000, -2.435693370351110282E-15, 21.50000000000000355 ) ) ;
#3402=ORIENTED_EDGE ( 'NONE', *, *, #5973, .T. ) ;
#3416=VERTEX_POINT ( 'NONE', #5830 ) ;
#3419=CIRCLE ( 'NONE', #5405, 0.7500000000000006661 ) ;
#3420=CARTESIAN_POINT ( 'NONE',  ( 0.7083562926195153819, -9.056472324687609543, -1.500000000000002887 ) ) ;
#3426=ORIENTED_EDGE ( 'NONE', *, *, #25169, .F. ) ;
#3434=VECTOR ( 'NONE', #28812, 1000.000000000000000 ) ;
#3441=DIRECTION ( 'NONE',  ( 0.000000000000000000, 1.132880637372608986E-16, -1.000000000000000000 ) ) ;
#3449=CARTESIAN_POINT ( 'NONE',  ( 7.488956955540398752, 5.141690706682901180, 21.50000000000000000 ) ) ;
#3456=EDGE_LOOP ( 'NONE', ( #12164, #17444, #17665, #3705 ) ) ;
#3458=CARTESIAN_POINT ( 'NONE',  ( 6.301234758012599357, -6.543385983536367689, 13.22130136205108819 ) ) ;
#3464=DIRECTION ( 'NONE',  ( 1.000000000000000000, 0.000000000000000000, 0.000000000000000000 ) ) ;
#3471=DIRECTION ( 'NONE',  ( 1.000000000000000000, 0.000000000000000000, 0.000000000000000000 ) ) ;
#3478=FACE_OUTER_BOUND ( 'NONE', #11529, .T. ) ;
#3488=EDGE_CURVE ( 'NONE', #19482, #29057, #16717, .T. ) ;
#3491=CARTESIAN_POINT ( 'NONE',  ( 1.492780340587499928E-15, -12.18947652193949693, 27.94260272410217638 ) ) ;
#3504=ADVANCED_FACE ( 'NONE', ( #5284 ), #2632, .F. ) ;
#3506=EDGE_CURVE ( 'NONE', #28205, #11519, #20211, .T. ) ;
#3509=EDGE_LOOP ( 'NONE', ( #9046, #22635 ) ) ;
#3530=VERTEX_POINT ( 'NONE', #12310 ) ;
#3539=CARTESIAN_POINT ( 'NONE',  ( 4.608906612435600181, 7.730328572437758616, -3.621320343559650379 ) ) ;
#3548=DIRECTION ( 'NONE',  ( 0.000000000000000000, 0.000000000000000000, 1.000000000000000000 ) ) ;
#3551=ORIENTED_EDGE ( 'NONE', *, *, #4438, .T. ) ;
#3553=CARTESIAN_POINT ( 'NONE',  ( -8.303920738747237351, -3.683253992019803746, 21.50000000000000000 ) ) ;
#3560=CARTESIAN_POINT ( 'NONE',  ( 8.999114229549594057, -0.1262659238204522361, 21.50000000000000000 ) ) ;
#3561=ORIENTED_EDGE ( 'NONE', *, *, #9780, .F. ) ;
#3577=ORIENTED_EDGE ( 'NONE', *, *, #8074, .T. ) ;
#3592=ORIENTED_EDGE ( 'NONE', *, *, #3131, .F. ) ;
#3606=AXIS2_PLACEMENT_3D ( 'NONE', #16561, #16417, #28123 ) ;
#3613=DIRECTION ( 'NONE',  ( -0.000000000000000000, -0.000000000000000000, 1.000000000000000000 ) ) ;
#3614=CARTESIAN_POINT ( 'NONE',  ( 2.516121109503181241, 8.728722367416590799, 21.50000000000000000 ) ) ;
#3638=DIRECTION ( 'NONE',  ( 0.000000000000000000, 1.000000000000000000, 0.000000000000000000 ) ) ;
#3643=CARTESIAN_POINT ( 'NONE',  ( 0.000000000000000000, -1.307826893540337417E-14, 27.94260272410217638 ) ) ;
#3654=CARTESIAN_POINT ( 'NONE',  ( -9.056472324687613096, -0.7083562926194845177, -1.500000000000001776 ) ) ;
#3664=EDGE_LOOP ( 'NONE', ( #19235, #27641, #25367 ) ) ;
#3668=ADVANCED_FACE ( 'NONE', ( #11364 ), #1840, .T. ) ;
#3682=CARTESIAN_POINT ( 'NONE',  ( -3.683253992019773992, 8.303920738747248009, 21.50000000000000000 ) ) ;
#3691=DIRECTION ( 'NONE',  ( 0.000000000000000000, 1.000000000000000000, 1.193512090021232842E-16 ) ) ;
#3699=VECTOR ( 'NONE', #21404, 1000.000000000000000 ) ;
#3705=ORIENTED_EDGE ( 'NONE', *, *, #14701, .T. ) ;
#3707=DIRECTION ( 'NONE',  ( -0.000000000000000000, 1.132880637372608986E-16, -1.000000000000000000 ) ) ;
#3726=DIRECTION ( 'NONE',  ( -0.000000000000000000, -0.000000000000000000, 1.000000000000000000 ) ) ;
#3728=CARTESIAN_POINT ( 'NONE',  ( -4.937793815610304726, 6.974883619896852238, 21.50000000000000000 ) ) ;
#3743=CARTESIAN_POINT ( 'NONE',  ( -2.446529495465445958, -8.413215745754985875, -3.621320343559650379 ) ) ;
#3744=VECTOR ( 'NONE', #4155, 1000.000000000000000 ) ;
#3750=DIRECTION ( 'NONE',  ( 0.000000000000000000, 0.000000000000000000, 1.000000000000000000 ) ) ;
#3752=CARTESIAN_POINT ( 'NONE',  ( -3.640207617113898841, 7.856594496258241023, 21.50000000000000000 ) ) ;
#3754=ORIENTED_EDGE ( 'NONE', *, *, #20621, .T. ) ;
#3781=PLANE ( 'NONE',  #3374 ) ;
#3789=DIRECTION ( 'NONE',  ( 0.000000000000000000, -1.132880637372608986E-16, 1.000000000000000000 ) ) ;
#3805=EDGE_CURVE ( 'NONE', #7334, #30279, #24208, .T. ) ;
#3807=VECTOR ( 'NONE', #18243, 1000.000000000000000 ) ;
#3810=LINE ( 'NONE', #10835, #25358 ) ;
#3813=CARTESIAN_POINT ( 'NONE',  ( 9.056472324687609543, 0.7083562926195455800, 21.50000000000000000 ) ) ;
#3816=AXIS2_PLACEMENT_3D ( 'NONE', #6664, #6522, #9022 ) ;
#3826=AXIS2_PLACEMENT_3D ( 'NONE', #8062, #5707, #3066 ) ;
#3835=PLANE ( 'NONE',  #25725 ) ;
#3857=VECTOR ( 'NONE', #16916, 1000.000000000000000 ) ;
#3887=ADVANCED_FACE ( 'NONE', ( #28653 ), #107, .T. ) ;
#3892=ORIENTED_EDGE ( 'NONE', *, *, #24207, .T. ) ;
#3902=AXIS2_PLACEMENT_3D ( 'NONE', #15016, #5981, #23416 ) ;
#3903=LINE ( 'NONE', #13426, #10959 ) ;
#3906=CARTESIAN_POINT ( 'NONE',  ( -4.390207617113899730, 7.856594496258241023, -1.500000000000000888 ) ) ;
#3909=EDGE_LOOP ( 'NONE', ( #753, #20312, #1916, #931 ) ) ;
#3911=EDGE_CURVE ( 'NONE', #18592, #5755, #29213, .T. ) ;
#3927=ORIENTED_EDGE ( 'NONE', *, *, #28055, .T. ) ;
#3946=AXIS2_PLACEMENT_3D ( 'NONE', #890, #1517, #24744 ) ;
#3961=AXIS2_PLACEMENT_3D ( 'NONE', #3539, #13203, #24900 ) ;
#3965=DIRECTION ( 'NONE',  ( 0.000000000000000000, 1.000000000000000000, 1.193512090021232842E-16 ) ) ;
#3980=DIRECTION ( 'NONE',  ( 1.000000000000000000, 0.000000000000000000, 0.000000000000000000 ) ) ;
#3982=DIRECTION ( 'NONE',  ( 1.000000000000000000, 0.000000000000000000, 0.000000000000000000 ) ) ;
#4005=( LENGTH_UNIT ( ) NAMED_UNIT ( * ) SI_UNIT ( .MILLI., .METRE. ) );
#4007=AXIS2_PLACEMENT_3D ( 'NONE', #504, #24192, #9867 ) ;
#4021=AXIS2_PLACEMENT_3D ( 'NONE', #17121, #3236, #12612 ) ;
#4041=CIRCLE ( 'NONE', #10515, 9.084132297865673777 ) ;
#4044=FACE_OUTER_BOUND ( 'NONE', #30217, .T. ) ;
#4051=CARTESIAN_POINT ( 'NONE',  ( 8.413215745754998309, -3.196529495465417980, 21.50000000000000000 ) ) ;
#4057=EDGE_CURVE ( 'NONE', #26463, #11295, #7281, .T. ) ;
#4081=EDGE_CURVE ( 'NONE', #1314, #25466, #15529, .T. ) ;
#4105=CARTESIAN_POINT ( 'NONE',  ( 8.752572334588123226, -2.431858781452763463, 21.50000000000000000 ) ) ;
#4121=VERTEX_POINT ( 'NONE', #13518 ) ;
#4128=ORIENTED_EDGE ( 'NONE', *, *, #4081, .T. ) ;
#4148=DIRECTION ( 'NONE',  ( 1.000000000000000000, 0.000000000000000000, 0.000000000000000000 ) ) ;
#4154=CARTESIAN_POINT ( 'NONE',  ( 6.974883619896790954, 5.687793815610376669, 21.50000000000000000 ) ) ;
#4155=DIRECTION ( 'NONE',  ( 0.000000000000000000, -1.132880637372608986E-16, 1.000000000000000000 ) ) ;
#4168=CYLINDRICAL_SURFACE ( 'NONE', #19812, 0.7500000000000006661 ) ;
#4176=CARTESIAN_POINT ( 'NONE',  ( 2.431858781452735041, 8.752572334588126779, 21.50000000000000000 ) ) ;
#4186=CARTESIAN_POINT ( 'NONE',  ( -9.056472324687611319, -0.7083562926194842957, 21.50000000000000000 ) ) ;
#4187=ORIENTED_EDGE ( 'NONE', *, *, #24263, .F. ) ;
#4191=CARTESIAN_POINT ( 'NONE',  ( -6.482337650448453559, -6.364020599487773211, 13.22130136205108819 ) ) ;
#4195=CARTESIAN_POINT ( 'NONE',  ( 5.687793815610356241, -6.974883619896809606, 21.50000000000000000 ) ) ;
#4203=EDGE_CURVE ( 'NONE', #7918, #25828, #27233, .T. ) ;
#4227=EDGE_CURVE ( 'NONE', #18904, #8467, #5218, .T. ) ;
#4243=LINE ( 'NONE', #5017, #7840 ) ;
#4248=DIRECTION ( 'NONE',  ( -0.000000000000000000, 1.132880637372608986E-16, -1.000000000000000000 ) ) ;
#4256=VERTEX_POINT ( 'NONE', #2878 ) ;
#4261=CYLINDRICAL_SURFACE ( 'NONE', #27545, 0.7500000000000006661 ) ;
#4263=CARTESIAN_POINT ( 'NONE',  ( -7.341751895053199028, 5.349779314757666882, 13.22130136205108819 ) ) ;
#4283=CIRCLE ( 'NONE', #19218, 9.084132297865673777 ) ;
#4293=ORIENTED_EDGE ( 'NONE', *, *, #15692, .F. ) ;
#4297=DIRECTION ( 'NONE',  ( 1.000000000000000000, 0.000000000000000000, 0.000000000000000000 ) ) ;
#4304=AXIS2_PLACEMENT_3D ( 'NONE', #19915, #17711, #10858 ) ;
#4305=DIRECTION ( 'NONE',  ( 1.000000000000000000, 0.000000000000000000, -0.000000000000000000 ) ) ;
#4306=VECTOR ( 'NONE', #20470, 1000.000000000000000 ) ;
#4310=DIRECTION ( 'NONE',  ( -0.000000000000000000, -0.000000000000000000, 1.000000000000000000 ) ) ;
#4315=AXIS2_PLACEMENT_3D ( 'NONE', #6599, #16415, #25927 ) ;
#4344=AXIS2_PLACEMENT_3D ( 'NONE', #4051, #13872, #23374 ) ;
#4367=FACE_OUTER_BOUND ( 'NONE', #20653, .T. ) ;
#4381=AXIS2_PLACEMENT_3D ( 'NONE', #25852, #16026, #23346 ) ;
#4387=EDGE_CURVE ( 'NONE', #7648, #29438, #22657, .T. ) ;
#4389=EDGE_CURVE ( 'NONE', #28571, #3416, #5320, .T. ) ;
#4397=ADVANCED_FACE ( 'NONE', ( #24540 ), #3188, .F. ) ;
#4407=AXIS2_PLACEMENT_3D ( 'NONE', #11659, #4639, #25700 ) ;
#4423=PLANE ( 'NONE',  #21066 ) ;
#4424=VERTEX_POINT ( 'NONE', #6456 ) ;
#4428=ORIENTED_EDGE ( 'NONE', *, *, #11577, .F. ) ;
#4430=PRODUCT ( 'Slotted Rotor Drive Shaft', 'Slotted Rotor Drive Shaft', '', ( #9606 ) ) ;
#4432=VECTOR ( 'NONE', #465, 1000.000000000000000 ) ;
#4434=EDGE_CURVE ( 'NONE', #9450, #2272, #25252, .T. ) ;
#4438=EDGE_CURVE ( 'NONE', #6357, #10933, #11798, .T. ) ;
#4451=LINE ( 'NONE', #16300, #1331 ) ;
#4460=CIRCLE ( 'NONE', #29856, 9.084132297865673777 ) ;
#4461=ORIENTED_EDGE ( 'NONE', *, *, #16791, .T. ) ;
#4464=EDGE_CURVE ( 'NONE', #20151, #29358, #14278, .T. ) ;
#4473=EDGE_CURVE ( 'NONE', #24171, #17300, #24729, .T. ) ;
#4482=CYLINDRICAL_SURFACE ( 'NONE', #18810, 0.7500000000000006661 ) ;
#4494=CIRCLE ( 'NONE', #7982, 0.7500000000000011102 ) ;
#4496=CARTESIAN_POINT ( 'NONE',  ( -5.881244434206279514, -6.812559277181949646, -3.621320343559650379 ) ) ;
#4497=VERTEX_POINT ( 'NONE', #22823 ) ;
#4503=DIRECTION ( 'NONE',  ( 1.156482317317871725E-15, 1.000000000000000000, 0.000000000000000000 ) ) ;
#4526=CARTESIAN_POINT ( 'NONE',  ( -8.840471615930058036, 1.687027447297517080, 21.50000000000000000 ) ) ;
#4535=CARTESIAN_POINT ( 'NONE',  ( -5.687793815610304726, 6.974883619896852238, -1.500000000000000888 ) ) ;
#4539=VERTEX_POINT ( 'NONE', #30151 ) ;
#4541=AXIS2_PLACEMENT_3D ( 'NONE', #7484, #27125, #5131 ) ;
#4546=DIRECTION ( 'NONE',  ( 1.000000000000000000, 0.000000000000000000, -0.000000000000000000 ) ) ;
#4565=AXIS2_PLACEMENT_3D ( 'NONE', #1195, #10700, #8213 ) ;
#4574=FACE_OUTER_BOUND ( 'NONE', #5111, .T. ) ;
#4585=CIRCLE ( 'NONE', #19020, 12.50000000000000000 ) ;
#4590=FACE_OUTER_BOUND ( 'NONE', #28756, .T. ) ;
#4596=CARTESIAN_POINT ( 'NONE',  ( 0.000000000000000000, -2.322405306613848348E-14, 117.5000000000000000 ) ) ;
#4598=DIRECTION ( 'NONE',  ( 1.000000000000000000, 0.000000000000000000, 0.000000000000000000 ) ) ;
#4605=ORIENTED_EDGE ( 'NONE', *, *, #27863, .F. ) ;
#4607=EDGE_CURVE ( 'NONE', #549, #30256, #7842, .T. ) ;
#4616=EDGE_CURVE ( 'NONE', #11338, #6047, #11733, .T. ) ;
#4628=DIRECTION ( 'NONE',  ( 1.000000000000000000, 0.000000000000000000, 0.000000000000000000 ) ) ;
#4632=CYLINDRICAL_SURFACE ( 'NONE', #23788, 0.7500000000000007772 ) ;
#4639=DIRECTION ( 'NONE',  ( 0.000000000000000000, 0.000000000000000000, 1.000000000000000000 ) ) ;
#4650=DIRECTION ( 'NONE',  ( 0.000000000000000000, 0.000000000000000000, 1.000000000000000000 ) ) ;
#4659=VECTOR ( 'NONE', #5520, 1000.000000000000000 ) ;
#4663=AXIS2_PLACEMENT_3D ( 'NONE', #29324, #7966, #26993 ) ;
#4686=CARTESIAN_POINT ( 'NONE',  ( -7.856594496258223259, -4.390207617113929039, 21.50000000000000000 ) ) ;
#4704=VECTOR ( 'NONE', #23050, 1000.000000000000000 ) ;
#4707=ORIENTED_EDGE ( 'NONE', *, *, #7500, .F. ) ;
#4711=VERTEX_POINT ( 'NONE', #14839 ) ;
#4717=ORIENTED_EDGE ( 'NONE', *, *, #21348, .F. ) ;
#4723=ORIENTED_EDGE ( 'NONE', *, *, #2706, .F. ) ;
#4741=ORIENTED_EDGE ( 'NONE', *, *, #25781, .T. ) ;
#4745=AXIS2_PLACEMENT_3D ( 'NONE', #14191, #2345, #10 ) ;
#4747=DIRECTION ( 'NONE',  ( 1.000000000000000000, 0.000000000000000000, 0.000000000000000000 ) ) ;
#4751=ORIENTED_EDGE ( 'NONE', *, *, #24059, .T. ) ;
#4767=AXIS2_PLACEMENT_3D ( 'NONE', #22328, #15298, #3464 ) ;
#4769=DIRECTION ( 'NONE',  ( -0.000000000000000000, 1.132880637372608986E-16, -1.000000000000000000 ) ) ;
#4778=LINE ( 'NONE', #259, #26740 ) ;
#4786=DIRECTION ( 'NONE',  ( 0.000000000000000000, -1.132880637372608986E-16, 1.000000000000000000 ) ) ;
#4793=DIRECTION ( 'NONE',  ( 0.000000000000000000, -1.132880637372608986E-16, 1.000000000000000000 ) ) ;
#4803=AXIS2_PLACEMENT_3D ( 'NONE', #7056, #16564, #19063 ) ;
#4807=CIRCLE ( 'NONE', #6391, 9.084132297865673777 ) ;
#4809=EDGE_LOOP ( 'NONE', ( #19388, #2819, #16274, #20379 ) ) ;
#4815=AXIS2_PLACEMENT_3D ( 'NONE', #4869, #14385, #23892 ) ;
#4829=DIRECTION ( 'NONE',  ( 0.000000000000000000, 0.000000000000000000, 1.000000000000000000 ) ) ;
#4834=DIRECTION ( 'NONE',  ( 1.000000000000000000, 0.000000000000000000, 0.000000000000000000 ) ) ;
#4839=AXIS2_PLACEMENT_3D ( 'NONE', #17881, #17705, #8057 ) ;
#4866=DIRECTION ( 'NONE',  ( -0.000000000000000000, -0.000000000000000000, 1.000000000000000000 ) ) ;
#4868=LINE ( 'NONE', #10593, #25520 ) ;
#4869=CARTESIAN_POINT ( 'NONE',  ( 0.1262659238204208167, 8.999114229549594057, -1.500000000000000888 ) ) ;
#4889=FACE_OUTER_BOUND ( 'NONE', #13109, .T. ) ;
#4899=ORIENTED_EDGE ( 'NONE', *, *, #24785, .F. ) ;
#4929=AXIS2_PLACEMENT_3D ( 'NONE', #6643, #16160, #4297 ) ;
#4953=ORIENTED_EDGE ( 'NONE', *, *, #21611, .T. ) ;
#4956=CARTESIAN_POINT ( 'NONE',  ( 6.543385983536345485, 6.301234758012618009, 13.22130136205108819 ) ) ;
#4966=CARTESIAN_POINT ( 'NONE',  ( -3.683253992019773992, 8.303920738747248009, 13.22130136205108997 ) ) ;
#4970=AXIS2_PLACEMENT_3D ( 'NONE', #6761, #9422, #25648 ) ;
#4986=ORIENTED_EDGE ( 'NONE', *, *, #13221, .F. ) ;
#5000=DIRECTION ( 'NONE',  ( 1.000000000000000000, 0.000000000000000000, 0.000000000000000000 ) ) ;
#5001=ADVANCED_FACE ( 'NONE', ( #28696 ), #30709, .F. ) ;
#5002=VERTEX_POINT ( 'NONE', #2764 ) ;
#5015=DIRECTION ( 'NONE',  ( 0.000000000000000000, 0.000000000000000000, 1.000000000000000000 ) ) ;
#5017=CARTESIAN_POINT ( 'NONE',  ( 1.112485354161228759E-15, -9.084132297865680883, 65.52304386563415051 ) ) ;
#5024=CARTESIAN_POINT ( 'NONE',  ( -8.752572334588105463, 2.431858781452820306, -1.500000000000001554 ) ) ;
#5026=ADVANCED_FACE ( 'NONE', ( #15061 ), #16950, .F. ) ;
#5027=CARTESIAN_POINT ( 'NONE',  ( -5.349779314757643789, -7.341751895053219457, 13.22130136205108819 ) ) ;
#5045=ORIENTED_EDGE ( 'NONE', *, *, #29382, .T. ) ;
#5063=ADVANCED_BREP_SHAPE_REPRESENTATION ( '', ( #2811, #7396 ), #11893 ) ;
#5085=CIRCLE ( 'NONE', #10565, 9.084132297865673777 ) ;
#5106=DIRECTION ( 'NONE',  ( 1.000000000000000000, 0.000000000000000000, 0.000000000000000000 ) ) ;
#5107=VERTEX_POINT ( 'NONE', #2920 ) ;
#5108=ORIENTED_EDGE ( 'NONE', *, *, #10925, .F. ) ;
#5111=EDGE_LOOP ( 'NONE', ( #12334, #25103 ) ) ;
#5131=DIRECTION ( 'NONE',  ( 1.000000000000000000, 0.000000000000000000, -0.000000000000000000 ) ) ;
#5143=PLANE ( 'NONE',  #2665 ) ;
#5152=DIRECTION ( 'NONE',  ( 0.000000000000000000, 0.000000000000000000, 1.000000000000000000 ) ) ;
#5158=FACE_OUTER_BOUND ( 'NONE', #14662, .T. ) ;
#5165=DIRECTION ( 'NONE',  ( 0.000000000000000000, -1.132880637372608986E-16, 1.000000000000000000 ) ) ;
#5167=CARTESIAN_POINT ( 'NONE',  ( 0.000000000000000000, 12.18947652193946851, 29.43090101791767665 ) ) ;
#5184=FACE_OUTER_BOUND ( 'NONE', #17156, .T. ) ;
#5192=EDGE_LOOP ( 'NONE', ( #14605, #10358 ) ) ;
#5203=AXIS2_PLACEMENT_3D ( 'NONE', #30843, #4650, #26327 ) ;
#5210=ORIENTED_EDGE ( 'NONE', *, *, #14701, .F. ) ;
#5214=DIRECTION ( 'NONE',  ( 1.000000000000000000, 0.000000000000000000, 0.000000000000000000 ) ) ;
#5218=LINE ( 'NONE', #2416, #23226 ) ;
#5234=CARTESIAN_POINT ( 'NONE',  ( -3.993622308618941741, -8.159193615868385763, 13.22130136205108641 ) ) ;
#5259=CARTESIAN_POINT ( 'NONE',  ( 6.301234758012599357, -6.543385983536367689, 21.50000000000000000 ) ) ;
#5261=ORIENTED_EDGE ( 'NONE', *, *, #25949, .T. ) ;
#5284=FACE_OUTER_BOUND ( 'NONE', #385, .T. ) ;
#5293=EDGE_LOOP ( 'NONE', ( #29784, #26572, #23619, #2932 ) ) ;
#5294=ORIENTED_EDGE ( 'NONE', *, *, #10365, .F. ) ;
#5298=FACE_OUTER_BOUND ( 'NONE', #20524, .T. ) ;
#5300=CIRCLE ( 'NONE', #23208, 0.7499999999999988898 ) ;
#5315=ORIENTED_EDGE ( 'NONE', *, *, #19878, .T. ) ;
#5320=CIRCLE ( 'NONE', #26749, 9.084132297865673777 ) ;
#5324=CARTESIAN_POINT ( 'NONE',  ( -8.134323311075783991, -1.438332125858144295, -1.500000000000001776 ) ) ;
#5352=ADVANCED_FACE ( 'NONE', ( #13200 ), #13054, .T. ) ;
#5353=EDGE_LOOP ( 'NONE', ( #729, #13270, #16495, #14119 ) ) ;
#5357=LINE ( 'NONE', #17364, #28800 ) ;
#5361=DIRECTION ( 'NONE',  ( 0.000000000000000000, -1.132880637372608986E-16, 1.000000000000000000 ) ) ;
#5380=VECTOR ( 'NONE', #12222, 1000.000000000000000 ) ;
#5398=CYLINDRICAL_SURFACE ( 'NONE', #17825, 0.7499999999999988898 ) ;
#5405=AXIS2_PLACEMENT_3D ( 'NONE', #22034, #21886, #17518 ) ;
#5406=CARTESIAN_POINT ( 'NONE',  ( 0.7083562926195156040, -9.056472324687613096, 21.50000000000000000 ) ) ;
#5423=VECTOR ( 'NONE', #3707, 1000.000000000000000 ) ;
#5424=ORIENTED_EDGE ( 'NONE', *, *, #21388, .F. ) ;
#5428=EDGE_CURVE ( 'NONE', #7702, #4497, #29782, .T. ) ;
#5452=EDGE_CURVE ( 'NONE', #30374, #4497, #2098, .T. ) ;
#5459=DIRECTION ( 'NONE',  ( 0.000000000000000000, -1.132880637372608986E-16, 1.000000000000000000 ) ) ;
#5500=DIRECTION ( 'NONE',  ( -0.000000000000000000, 1.132880637372608986E-16, -1.000000000000000000 ) ) ;
#5508=CIRCLE ( 'NONE', #4021, 0.7499999999999997780 ) ;
#5520=DIRECTION ( 'NONE',  ( 0.000000000000000000, -1.132880637372608986E-16, 1.000000000000000000 ) ) ;
#5521=ORIENTED_EDGE ( 'NONE', *, *, #26339, .T. ) ;
#5572=ORIENTED_EDGE ( 'NONE', *, *, #4607, .F. ) ;
#5578=ORIENTED_EDGE ( 'NONE', *, *, #7927, .F. ) ;
#5586=CARTESIAN_POINT ( 'NONE',  ( 0.9621688436939442868, 9.033033306777458193, 13.22130136205108997 ) ) ;
#5587=CYLINDRICAL_SURFACE ( 'NONE', #1533, 0.7500000000000006661 ) ;
#5593=ORIENTED_EDGE ( 'NONE', *, *, #17182, .F. ) ;
#5599=CARTESIAN_POINT ( 'NONE',  ( -5.141690706682821244, 7.488956955540452043, 21.50000000000000000 ) ) ;
#5607=ORIENTED_EDGE ( 'NONE', *, *, #19301, .F. ) ;
#5618=AXIS2_PLACEMENT_3D ( 'NONE', #11663, #9171, #18683 ) ;
#5621=DIRECTION ( 'NONE',  ( 0.000000000000000000, 0.000000000000000000, 1.000000000000000000 ) ) ;
#5622=CARTESIAN_POINT ( 'NONE',  ( -5.349779314757643789, -7.341751895053219457, 21.50000000000000000 ) ) ;
#5624=ORIENTED_EDGE ( 'NONE', *, *, #15656, .F. ) ;
#5631=ADVANCED_FACE ( 'NONE', ( #11585 ), #25486, .F. ) ;
#5633=ADVANCED_FACE ( 'NONE', ( #11735 ), #30758, .T. ) ;
#5644=ORIENTED_EDGE ( 'NONE', *, *, #23523, .T. ) ;
#5658=DIRECTION ( 'NONE',  ( 0.000000000000000000, -1.000000000000000000, -1.132880637372608986E-16 ) ) ;
#5669=AXIS2_PLACEMENT_3D ( 'NONE', #742, #3245, #15094 ) ;
#5670=CARTESIAN_POINT ( 'NONE',  ( -4.390207617113899730, 7.856594496258241023, -1.500000000000000888 ) ) ;
#5676=ORIENTED_EDGE ( 'NONE', *, *, #2539, .T. ) ;
#5684=ORIENTED_EDGE ( 'NONE', *, *, #19878, .F. ) ;
#5692=DIRECTION ( 'NONE',  ( 1.000000000000000000, 0.000000000000000000, 0.000000000000000000 ) ) ;
#5693=VECTOR ( 'NONE', #18548, 1000.000000000000000 ) ;
#5695=FACE_OUTER_BOUND ( 'NONE', #2785, .T. ) ;
#5699=DIRECTION ( 'NONE',  ( 0.000000000000000000, -1.132880637372608986E-16, 1.000000000000000000 ) ) ;
#5707=DIRECTION ( 'NONE',  ( 0.000000000000000000, -1.132880637372608986E-16, 1.000000000000000000 ) ) ;
#5724=ADVANCED_FACE ( 'NONE', ( #21227 ), #2374, .F. ) ;
#5726=ORIENTED_EDGE ( 'NONE', *, *, #9575, .T. ) ;
#5737=ADVANCED_FACE ( 'NONE', ( #21078 ), #9242, .F. ) ;
#5739=EDGE_LOOP ( 'NONE', ( #26528, #21334, #18292, #19438 ) ) ;
#5749=DIRECTION ( 'NONE',  ( 1.000000000000000000, 0.000000000000000000, 0.000000000000000000 ) ) ;
#5753=CARTESIAN_POINT ( 'NONE',  ( -8.817355867515827228, -2.185336383880175593, -1.500000000000001998 ) ) ;
#5755=VERTEX_POINT ( 'NONE', #5024 ) ;
#5756=VERTEX_POINT ( 'NONE', #22590 ) ;
#5773=ORIENTED_EDGE ( 'NONE', *, *, #23301, .T. ) ;
#5775=VERTEX_POINT ( 'NONE', #24937 ) ;
#5787=CIRCLE ( 'NONE', #12758, 7.500000000000007105 ) ;
#5798=CARTESIAN_POINT ( 'NONE',  ( 2.185336383880204014, -8.817355867515821899, 21.50000000000000000 ) ) ;
#5805=DIRECTION ( 'NONE',  ( 0.000000000000000000, 0.000000000000000000, 1.000000000000000000 ) ) ;
#5809=ORIENTED_EDGE ( 'NONE', *, *, #6087, .T. ) ;
#5810=VECTOR ( 'NONE', #13804, 1000.000000000000000 ) ;
#5811=AXIS2_PLACEMENT_3D ( 'NONE', #13385, #6354, #8697 ) ;
#5819=EDGE_LOOP ( 'NONE', ( #7696, #14472 ) ) ;
#5820=FACE_OUTER_BOUND ( 'NONE', #7033, .T. ) ;
#5823=CYLINDRICAL_SURFACE ( 'NONE', #29449, 0.7499999999999997780 ) ;
#5830=CARTESIAN_POINT ( 'NONE',  ( 8.159193615868398197, -3.993622308618910210, -1.500000000000002220 ) ) ;
#5832=ORIENTED_EDGE ( 'NONE', *, *, #19927, .T. ) ;
#5844=ORIENTED_EDGE ( 'NONE', *, *, #29402, .T. ) ;
#5849=VERTEX_POINT ( 'NONE', #3420 ) ;
#5850=DIRECTION ( 'NONE',  ( 0.000000000000000000, 1.132880637372608986E-16, -1.000000000000000000 ) ) ;
#5857=EDGE_LOOP ( 'NONE', ( #903, #26096 ) ) ;
#5859=VECTOR ( 'NONE', #10010, 1000.000000000000000 ) ;
#5860=AXIS2_PLACEMENT_3D ( 'NONE', #9198, #16836, #21179 ) ;
#5868=CIRCLE ( 'NONE', #23288, 9.084132297865673777 ) ;
#5883=( NAMED_UNIT ( * ) PLANE_ANGLE_UNIT ( ) SI_UNIT ( $, .RADIAN. ) );
#5886=AXIS2_PLACEMENT_3D ( 'NONE', #19328, #12479, #23989 ) ;
#5893=CARTESIAN_POINT ( 'NONE',  ( -4.608906612435655248, -7.730328572437724866, -3.621320343559650379 ) ) ;
#5904=CIRCLE ( 'NONE', #13875, 9.084132297865673777 ) ;
#5907=EDGE_CURVE ( 'NONE', #21461, #9461, #4868, .T. ) ;
#5920=EDGE_CURVE ( 'NONE', #16597, #19689, #29504, .T. ) ;
#5927=DIRECTION ( 'NONE',  ( 0.000000000000000000, 0.000000000000000000, 1.000000000000000000 ) ) ;
#5929=AXIS2_PLACEMENT_3D ( 'NONE', #30799, #23461, #20668 ) ;
#5941=ORIENTED_EDGE ( 'NONE', *, *, #18725, .T. ) ;
#5948=CYLINDRICAL_SURFACE ( 'NONE', #28791, 0.7499999999999997780 ) ;
#5960=DIRECTION ( 'NONE',  ( 0.000000000000000000, 0.000000000000000000, 1.000000000000000000 ) ) ;
#5963=DIRECTION ( 'NONE',  ( 0.000000000000000000, 1.132880637372608986E-16, -1.000000000000000000 ) ) ;
#5973=EDGE_CURVE ( 'NONE', #897, #27328, #8113, .T. ) ;
#5981=DIRECTION ( 'NONE',  ( 0.000000000000000000, -1.132880637372608986E-16, 1.000000000000000000 ) ) ;
#5988=ADVANCED_FACE ( 'NONE', ( #7143 ), #6987, .F. ) ;
#5991=ADVANCED_FACE ( 'NONE', ( #21008 ), #14005, .F. ) ;
#6011=ADVANCED_FACE ( 'NONE', ( #28190 ), #28661, .F. ) ;
#6012=CARTESIAN_POINT ( 'NONE',  ( 8.999114229549594057, -0.1262659238204522361, -3.621320343559650379 ) ) ;
#6021=CARTESIAN_POINT ( 'NONE',  ( 0.000000000000000000, -2.322405306613848348E-14, 117.5000000000000000 ) ) ;
#6034=DIRECTION ( 'NONE',  ( 1.000000000000000000, 0.000000000000000000, -0.000000000000000000 ) ) ;
#6045=VERTEX_POINT ( 'NONE', #28364 ) ;
#6047=VERTEX_POINT ( 'NONE', #16497 ) ;
#6066=EDGE_LOOP ( 'NONE', ( #5644, #20685, #8967, #4187 ) ) ;
#6070=VERTEX_POINT ( 'NONE', #21318 ) ;
#6074=ORIENTED_EDGE ( 'NONE', *, *, #19110, .F. ) ;
#6076=CARTESIAN_POINT ( 'NONE',  ( 0.1262659238204208167, 8.999114229549594057, 21.50000000000000000 ) ) ;
#6083=ORIENTED_EDGE ( 'NONE', *, *, #1549, .F. ) ;
#6087=EDGE_CURVE ( 'NONE', #26020, #3416, #26159, .T. ) ;
#6109=DIRECTION ( 'NONE',  ( 1.000000000000000000, 0.000000000000000000, 0.000000000000000000 ) ) ;
#6130=CARTESIAN_POINT ( 'NONE',  ( 8.499586724479435418, 2.959227181723830036, -1.500000000000001332 ) ) ;
#6131=CARTESIAN_POINT ( 'NONE',  ( 5.687793815610356241, -6.974883619896809606, -3.621320343559650379 ) ) ;
#6150=PLANE ( 'NONE',  #15055 ) ;
#6151=ORIENTED_EDGE ( 'NONE', *, *, #19904, .T. ) ;
#6160=CARTESIAN_POINT ( 'NONE',  ( -0.9370274472974918778, -8.840471615930066918, -1.500000000000002665 ) ) ;
#6180=CARTESIAN_POINT ( 'NONE',  ( 0.000000000000000000, -2.435693370351110282E-15, 21.50000000000000355 ) ) ;
#6183=CARTESIAN_POINT ( 'NONE',  ( 0.000000000000000000, 0.000000000000000000, -87.50000000000000000 ) ) ;
#6186=DIRECTION ( 'NONE',  ( 0.000000000000000000, 0.000000000000000000, 1.000000000000000000 ) ) ;
#6203=VERTEX_POINT ( 'NONE', #24283 ) ;
#6218=DIRECTION ( 'NONE',  ( 1.000000000000000000, 0.000000000000000000, 0.000000000000000000 ) ) ;
#6231=VERTEX_POINT ( 'NONE', #3074 ) ;
#6237=ORIENTED_EDGE ( 'NONE', *, *, #29402, .F. ) ;
#6258=PLANE ( 'NONE',  #29286 ) ;
#6263=DIRECTION ( 'NONE',  ( 1.000000000000000000, 0.000000000000000000, 0.000000000000000000 ) ) ;
#6275=ORIENTED_EDGE ( 'NONE', *, *, #27609, .T. ) ;
#6286=AXIS2_PLACEMENT_3D ( 'NONE', #10030, #19537, #12530 ) ;
#6302=DIRECTION ( 'NONE',  ( 0.000000000000000000, -1.132880637372608986E-16, 1.000000000000000000 ) ) ;
#6309=EDGE_CURVE ( 'NONE', #29624, #18134, #20826, .T. ) ;
#6311=DIRECTION ( 'NONE',  ( 0.000000000000000000, 1.000000000000000000, 1.193512090021232842E-16 ) ) ;
#6318=CARTESIAN_POINT ( 'NONE',  ( 3.914781618004695929, 8.197313248159961319, -1.500000000000000888 ) ) ;
#6322=DIRECTION ( 'NONE',  ( -0.000000000000000000, 1.132880637372608986E-16, -1.000000000000000000 ) ) ;
#6334=AXIS2_PLACEMENT_3D ( 'NONE', #26539, #7364, #14373 ) ;
#6338=AXIS2_PLACEMENT_3D ( 'NONE', #21928, #557, #10077 ) ;
#6343=ORIENTED_EDGE ( 'NONE', *, *, #21967, .T. ) ;
#6348=ADVANCED_FACE ( 'NONE', ( #23159 ), #13209, .T. ) ;
#6353=CIRCLE ( 'NONE', #29779, 9.084132297865673777 ) ;
#6354=DIRECTION ( 'NONE',  ( 0.000000000000000000, 1.132880637372608986E-16, -1.000000000000000000 ) ) ;
#6357=VERTEX_POINT ( 'NONE', #15685 ) ;
#6368=ADVANCED_FACE ( 'NONE', ( #13368 ), #11021, .F. ) ;
#6375=CYLINDRICAL_SURFACE ( 'NONE', #16367, 0.7500000000000011102 ) ;
#6376=ORIENTED_EDGE ( 'NONE', *, *, #19964, .F. ) ;
#6383=ORIENTED_EDGE ( 'NONE', *, *, #1790, .T. ) ;
#6388=LINE ( 'NONE', #13566, #20051 ) ;
#6389=CIRCLE ( 'NONE', #30773, 9.084132297865673777 ) ;
#6391=AXIS2_PLACEMENT_3D ( 'NONE', #6593, #15958, #16247 ) ;
#6393=ORIENTED_EDGE ( 'NONE', *, *, #25579, .T. ) ;
#6411=ORIENTED_EDGE ( 'NONE', *, *, #16063, .F. ) ;
#6424=CARTESIAN_POINT ( 'NONE',  ( -2.516121109503243414, -8.728722367416578365, 13.22130136205108641 ) ) ;
#6435=DIRECTION ( 'NONE',  ( 0.000000000000000000, -1.132880637372608986E-16, 1.000000000000000000 ) ) ;
#6450=DIRECTION ( 'NONE',  ( 0.000000000000000000, 1.000000000000000000, 0.000000000000000000 ) ) ;
#6455=CARTESIAN_POINT ( 'NONE',  ( 0.000000000000000000, -2.435693370351110282E-15, 21.50000000000000355 ) ) ;
#6456=CARTESIAN_POINT ( 'NONE',  ( 6.543385983536345485, 6.301234758012618009, 21.50000000000000000 ) ) ;
#6457=DIRECTION ( 'NONE',  ( 1.000000000000000000, 0.000000000000000000, 0.000000000000000000 ) ) ;
#6462=ORIENTED_EDGE ( 'NONE', *, *, #12893, .T. ) ;
#6470=ORIENTED_EDGE ( 'NONE', *, *, #24313, .T. ) ;
#6502=LINE ( 'NONE', #16011, #3744 ) ;
#6512=EDGE_CURVE ( 'NONE', #30374, #9285, #18084, .T. ) ;
#6516=ORIENTED_EDGE ( 'NONE', *, *, #28292, .T. ) ;
#6522=DIRECTION ( 'NONE',  ( -0.000000000000000000, 1.132880637372608986E-16, -1.000000000000000000 ) ) ;
#6523=DIRECTION ( 'NONE',  ( 0.000000000000000000, 0.000000000000000000, 1.000000000000000000 ) ) ;
#6539=CARTESIAN_POINT ( 'NONE',  ( 0.000000000000000000, 1.699320956058915452E-16, -1.500000000000001776 ) ) ;
#6542=DIRECTION ( 'NONE',  ( 2.312964634635740689E-15, 1.000000000000000000, 0.000000000000000000 ) ) ;
#6543=ORIENTED_EDGE ( 'NONE', *, *, #14321, .F. ) ;
#6544=DIRECTION ( 'NONE',  ( -0.000000000000000000, 1.132880637372608986E-16, -1.000000000000000000 ) ) ;
#6545=ADVANCED_FACE ( 'NONE', ( #7878 ), #533, .F. ) ;
#6551=ORIENTED_EDGE ( 'NONE', *, *, #25767, .T. ) ;
#6593=CARTESIAN_POINT ( 'NONE',  ( 0.000000000000000000, 1.699320956058915452E-16, -1.500000000000001776 ) ) ;
#6596=DIRECTION ( 'NONE',  ( 1.000000000000000000, 0.000000000000000000, 0.000000000000000000 ) ) ;
#6599=CARTESIAN_POINT ( 'NONE',  ( 1.687027447297431371, 8.840471615930075799, -1.500000000000000888 ) ) ;
#6601=DIRECTION ( 'NONE',  ( -0.000000000000000000, -0.000000000000000000, 1.000000000000000000 ) ) ;
#6627=CIRCLE ( 'NONE', #22071, 0.7500000000000002220 ) ;
#6629=CARTESIAN_POINT ( 'NONE',  ( 8.840471615930072247, -1.687027447297460236, -3.621320343559650379 ) ) ;
#6638=DIRECTION ( 'NONE',  ( -0.000000000000000000, 1.132880637372608986E-16, -1.000000000000000000 ) ) ;
#6640=EDGE_LOOP ( 'NONE', ( #2948, #13993, #21064, #103 ) ) ;
#6643=CARTESIAN_POINT ( 'NONE',  ( -1.687027447297492211, -8.840471615930066918, 21.50000000000000000 ) ) ;
#6659=CARTESIAN_POINT ( 'NONE',  ( -8.499586724479453181, -2.959227181723774525, -3.621320343559650379 ) ) ;
#6664=CARTESIAN_POINT ( 'NONE',  ( 0.000000000000000000, 0.000000000000000000, -87.50000000000000000 ) ) ;
#6668=CARTESIAN_POINT ( 'NONE',  ( 0.000000000000000000, -2.435693370351110282E-15, 21.50000000000000355 ) ) ;
#6677=ADVANCED_FACE ( 'NONE', ( #3039 ), #19416, .F. ) ;
#6687=CARTESIAN_POINT ( 'NONE',  ( 0.8762659238204211221, 8.999114229549594057, -1.500000000000000888 ) ) ;
#6705=ORIENTED_EDGE ( 'NONE', *, *, #4438, .F. ) ;
#6711=EDGE_CURVE ( 'NONE', #17300, #6047, #25560, .T. ) ;
#6713=LINE ( 'NONE', #9210, #11369 ) ;
#6724=ADVANCED_FACE ( 'NONE', ( #29870 ), #29548, .F. ) ;
#6740=CARTESIAN_POINT ( 'NONE',  ( 8.728722367416583694, -2.516121109503213216, 13.22130136205108819 ) ) ;
#6758=VERTEX_POINT ( 'NONE', #15340 ) ;
#6761=CARTESIAN_POINT ( 'NONE',  ( 0.000000000000000000, -2.775557561562891351E-14, 157.4999999999999716 ) ) ;
#6772=CARTESIAN_POINT ( 'NONE',  ( 8.795879380940563763, 2.270234684139707859, -1.500000000000001554 ) ) ;
#6820=AXIS2_PLACEMENT_3D ( 'NONE', #7674, #2997, #12357 ) ;
#6824=VERTEX_POINT ( 'NONE', #21234 ) ;
#6829=AXIS2_PLACEMENT_3D ( 'NONE', #24427, #19445, #26468 ) ;
#6835=AXIS2_PLACEMENT_3D ( 'NONE', #22917, #3750, #1565 ) ;
#6836=DIRECTION ( 'NONE',  ( 0.000000000000000000, 1.000000000000000000, 1.156482317317869999E-16 ) ) ;
#6851=DIRECTION ( 'NONE',  ( -1.243218491116710699E-14, 1.000000000000000000, 0.000000000000000000 ) ) ;
#6865=FACE_OUTER_BOUND ( 'NONE', #30544, .T. ) ;
#6869=EDGE_CURVE ( 'NONE', #9137, #26641, #23427, .T. ) ;
#6870=DIRECTION ( 'NONE',  ( 1.000000000000000000, 0.000000000000000000, 0.000000000000000000 ) ) ;
#6880=EDGE_LOOP ( 'NONE', ( #2481, #17859, #18852 ) ) ;
#6884=ORIENTED_EDGE ( 'NONE', *, *, #22415, .F. ) ;
#6887=LINE ( 'NONE', #11888, #23727 ) ;
#6889=DIRECTION ( 'NONE',  ( 0.000000000000000000, 0.000000000000000000, 1.000000000000000000 ) ) ;
#6892=DIRECTION ( 'NONE',  ( 0.000000000000000000, 0.000000000000000000, 1.000000000000000000 ) ) ;
#6899=CIRCLE ( 'NONE', #13378, 0.7500000000000006661 ) ;
#6901=LINE ( 'NONE', #22967, #20807 ) ;
#6906=CARTESIAN_POINT ( 'NONE',  ( 1.438332125858173605, -8.884323311075778662, 21.50000000000000000 ) ) ;
#6908=LINE ( 'NONE', #7055, #27693 ) ;
#6913=ORIENTED_EDGE ( 'NONE', *, *, #24096, .T. ) ;
#6918=FACE_OUTER_BOUND ( 'NONE', #5739, .T. ) ;
#6919=VERTEX_POINT ( 'NONE', #25133 ) ;
#6921=DIRECTION ( 'NONE',  ( 0.000000000000000000, 0.000000000000000000, 1.000000000000000000 ) ) ;
#6947=CARTESIAN_POINT ( 'NONE',  ( -0.7083562926194498788, 9.056472324687613096, 21.50000000000000000 ) ) ;
#6966=EDGE_CURVE ( 'NONE', #28599, #10212, #21554, .T. ) ;
#6972=DIRECTION ( 'NONE',  ( 0.000000000000000000, 0.000000000000000000, 1.000000000000000000 ) ) ;
#6985=ORIENTED_EDGE ( 'NONE', *, *, #8447, .F. ) ;
#6987=CYLINDRICAL_SURFACE ( 'NONE', #29027, 0.7500000000000006661 ) ;
#6993=CARTESIAN_POINT ( 'NONE',  ( -3.993622308618941741, -8.159193615868385763, 21.50000000000000000 ) ) ;
#6994=EDGE_LOOP ( 'NONE', ( #29128, #11345, #20847, #5572 ) ) ;
#6998=EDGE_CURVE ( 'NONE', #2547, #6824, #13296, .T. ) ;
#7026=LINE ( 'NONE', #28241, #25863 ) ;
#7030=CARTESIAN_POINT ( 'NONE',  ( 0.9621688436939443978, 9.033033306777458193, 21.50000000000000000 ) ) ;
#7033=EDGE_LOOP ( 'NONE', ( #9419, #5578 ) ) ;
#7041=DIRECTION ( 'NONE',  ( 0.000000000000000000, 0.000000000000000000, 1.000000000000000000 ) ) ;
#7042=DIRECTION ( 'NONE',  ( -0.000000000000000000, -0.000000000000000000, 1.000000000000000000 ) ) ;
#7055=CARTESIAN_POINT ( 'NONE',  ( -3.858906612435654804, -7.730328572437724866, -3.621320343559650379 ) ) ;
#7056=CARTESIAN_POINT ( 'NONE',  ( -8.884323311075783991, -1.438332125858144295, -1.500000000000001776 ) ) ;
#7059=ORIENTED_EDGE ( 'NONE', *, *, #4057, .T. ) ;
#7064=DIRECTION ( 'NONE',  ( -0.000000000000000000, -0.000000000000000000, 1.000000000000000000 ) ) ;
#7066=CARTESIAN_POINT ( 'NONE',  ( 0.000000000000000000, 1.699320956058915452E-16, -1.500000000000001776 ) ) ;
#7077=ORIENTED_EDGE ( 'NONE', *, *, #11266, .T. ) ;
#7082=CIRCLE ( 'NONE', #13019, 0.7500000000000006661 ) ;
#7106=EDGE_CURVE ( 'NONE', #6203, #699, #17114, .T. ) ;
#7123=VECTOR ( 'NONE', #8244, 1000.000000000000000 ) ;
#7126=LINE ( 'NONE', #11795, #9071 ) ;
#7139=VERTEX_POINT ( 'NONE', #15940 ) ;
#7143=FACE_OUTER_BOUND ( 'NONE', #688, .T. ) ;
#7156=ORIENTED_EDGE ( 'NONE', *, *, #5428, .T. ) ;
#7162=AXIS2_PLACEMENT_3D ( 'NONE', #17864, #18323, #22668 ) ;
#7170=CARTESIAN_POINT ( 'NONE',  ( -8.197313248159920462, 3.914781618004780306, 13.22130136205108819 ) ) ;
#7173=EDGE_LOOP ( 'NONE', ( #5593, #28664, #26099, #21695 ) ) ;
#7187=DIRECTION ( 'NONE',  ( 1.000000000000000000, 0.000000000000000000, 0.000000000000000000 ) ) ;
#7189=FACE_OUTER_BOUND ( 'NONE', #18774, .T. ) ;
#7190=ORIENTED_EDGE ( 'NONE', *, *, #28306, .F. ) ;
#7198=CIRCLE ( 'NONE', #16158, 0.7500000000000006661 ) ;
#7204=CARTESIAN_POINT ( 'NONE',  ( 0.000000000000000000, -2.322405306613848348E-14, 117.5000000000000000 ) ) ;
#7209=CYLINDRICAL_SURFACE ( 'NONE', #7312, 0.7500000000000011102 ) ;
#7211=VERTEX_POINT ( 'NONE', #16533 ) ;
#7222=EDGE_LOOP ( 'NONE', ( #2950, #29909 ) ) ;
#7228=CARTESIAN_POINT ( 'NONE',  ( 0.000000000000000000, 1.699320956058915452E-16, -1.500000000000001776 ) ) ;
#7239=FACE_OUTER_BOUND ( 'NONE', #3456, .T. ) ;
#7268=CARTESIAN_POINT ( 'NONE',  ( 0.000000000000000000, 1.699320956058915452E-16, -1.500000000000001776 ) ) ;
#7271=CIRCLE ( 'NONE', #22689, 0.7500000000000004441 ) ;
#7273=ORIENTED_EDGE ( 'NONE', *, *, #25991, .T. ) ;
#7280=DIRECTION ( 'NONE',  ( 0.000000000000000000, -1.132880637372608986E-16, 1.000000000000000000 ) ) ;
#7281=CIRCLE ( 'NONE', #24709, 15.00000000000003553 ) ;
#7283=DIRECTION ( 'NONE',  ( 0.000000000000000000, -1.132880637372608986E-16, 1.000000000000000000 ) ) ;
#7295=EDGE_CURVE ( 'NONE', #25948, #8229, #22072, .T. ) ;
#7312=AXIS2_PLACEMENT_3D ( 'NONE', #24190, #26235, #12364 ) ;
#7318=ADVANCED_FACE ( 'NONE', ( #5298 ), #5143, .F. ) ;
#7320=CIRCLE ( 'NONE', #13779, 0.7500000000000006661 ) ;
#7334=VERTEX_POINT ( 'NONE', #26200 ) ;
#7338=PLANE ( 'NONE',  #24308 ) ;
#7352=ORIENTED_EDGE ( 'NONE', *, *, #2529, .T. ) ;
#7364=DIRECTION ( 'NONE',  ( -0.000000000000000000, 1.132880637372608986E-16, -1.000000000000000000 ) ) ;
#7365=CIRCLE ( 'NONE', #28776, 9.084132297865673777 ) ;
#7370=DIRECTION ( 'NONE',  ( 0.000000000000000000, 1.000000000000000000, 0.000000000000000000 ) ) ;
#7396=AXIS2_PLACEMENT_3D ( 'NONE', #9486, #28514, #21014 ) ;
#7398=CARTESIAN_POINT ( 'NONE',  ( 0.000000000000000000, 1.699320956058915452E-16, -1.500000000000001776 ) ) ;
#7408=CARTESIAN_POINT ( 'NONE',  ( -2.209227181723746103, 8.499586724479465616, -3.621320343559650379 ) ) ;
#7418=ORIENTED_EDGE ( 'NONE', *, *, #9001, .F. ) ;
#7419=DIRECTION ( 'NONE',  ( 0.000000000000000000, 1.000000000000000000, 0.000000000000000000 ) ) ;
#7434=CARTESIAN_POINT ( 'NONE',  ( 9.056472324687607767, 0.7083562926195451359, -1.500000000000001776 ) ) ;
#7472=ORIENTED_EDGE ( 'NONE', *, *, #22914, .T. ) ;
#7473=EDGE_CURVE ( 'NONE', #11838, #17742, #16598, .T. ) ;
#7479=AXIS2_PLACEMENT_3D ( 'NONE', #10559, #29736, #11176 ) ;
#7484=CARTESIAN_POINT ( 'NONE',  ( 8.999114229549594057, -0.1262659238204522361, 21.50000000000000000 ) ) ;
#7497=EDGE_CURVE ( 'NONE', #22829, #23519, #14578, .T. ) ;
#7500=EDGE_CURVE ( 'NONE', #16268, #11562, #27035, .T. ) ;
#7506=ORIENTED_EDGE ( 'NONE', *, *, #27881, .F. ) ;
#7521=PLANE ( 'NONE',  #15807 ) ;
#7523=ORIENTED_EDGE ( 'NONE', *, *, #376, .F. ) ;
#7530=DIRECTION ( 'NONE',  ( -0.000000000000000000, 1.132880637372608986E-16, -1.000000000000000000 ) ) ;
#7540=DIRECTION ( 'NONE',  ( 1.000000000000000000, 0.000000000000000000, -0.000000000000000000 ) ) ;
#7545=ORIENTED_EDGE ( 'NONE', *, *, #20976, .T. ) ;
#7554=VERTEX_POINT ( 'NONE', #15905 ) ;
#7568=EDGE_CURVE ( 'NONE', #24166, #1662, #30079, .T. ) ;
#7589=DIRECTION ( 'NONE',  ( 0.000000000000000000, 1.132880637372608986E-16, -1.000000000000000000 ) ) ;
#7602=ORIENTED_EDGE ( 'NONE', *, *, #26210, .T. ) ;
#7620=ORIENTED_EDGE ( 'NONE', *, *, #11084, .F. ) ;
#7621=DIRECTION ( 'NONE',  ( 0.000000000000000000, -1.132880637372608986E-16, 1.000000000000000000 ) ) ;
#7628=PLANE ( 'NONE',  #4541 ) ;
#7629=FACE_OUTER_BOUND ( 'NONE', #24715, .T. ) ;
#7643=DIRECTION ( 'NONE',  ( 1.000000000000000000, 0.000000000000000000, -0.000000000000000000 ) ) ;
#7648=VERTEX_POINT ( 'NONE', #30088 ) ;
#7649=CIRCLE ( 'NONE', #5669, 0.7500000000000006661 ) ;
#7652=CARTESIAN_POINT ( 'NONE',  ( 0.000000000000000000, 1.699320956058915452E-16, -1.500000000000001776 ) ) ;
#7655=EDGE_CURVE ( 'NONE', #20169, #11001, #6388, .T. ) ;
#7656=CARTESIAN_POINT ( 'NONE',  ( 3.196529495465388226, 8.413215745755008967, 21.50000000000000000 ) ) ;
#7662=FACE_OUTER_BOUND ( 'NONE', #27843, .T. ) ;
#7673=EDGE_CURVE ( 'NONE', #26525, #22829, #21445, .T. ) ;
#7674=CARTESIAN_POINT ( 'NONE',  ( 0.000000000000000000, -2.435693370351110282E-15, 21.50000000000000355 ) ) ;
#7693=CARTESIAN_POINT ( 'NONE',  ( 7.341751895053238108, -5.349779314757616255, 13.22130136205108819 ) ) ;
#7695=CARTESIAN_POINT ( 'NONE',  ( 8.840471615930072247, -1.687027447297460236, 21.50000000000000000 ) ) ;
#7696=ORIENTED_EDGE ( 'NONE', *, *, #13398, .F. ) ;
#7702=VERTEX_POINT ( 'NONE', #22058 ) ;
#7706=AXIS2_PLACEMENT_3D ( 'NONE', #11030, #13381, #15696 ) ;
#7713=VERTEX_POINT ( 'NONE', #15036 ) ;
#7717=CARTESIAN_POINT ( 'NONE',  ( 9.056472324687607767, 0.7083562926195454690, 13.22130136205108819 ) ) ;
#7719=ORIENTED_EDGE ( 'NONE', *, *, #11645, .T. ) ;
#7720=LINE ( 'NONE', #7408, #3857 ) ;
#7731=FACE_OUTER_BOUND ( 'NONE', #5293, .T. ) ;
#7821=DIRECTION ( 'NONE',  ( 0.000000000000000000, 0.000000000000000000, 1.000000000000000000 ) ) ;
#7823=ORIENTED_EDGE ( 'NONE', *, *, #7673, .T. ) ;
#7824=DIRECTION ( 'NONE',  ( 0.000000000000000000, 0.000000000000000000, 1.000000000000000000 ) ) ;
#7830=ADVANCED_FACE ( 'NONE', ( #16126, #13177 ), #6150, .T. ) ;
#7840=VECTOR ( 'NONE', #23564, 1000.000000000000000 ) ;
#7842=CIRCLE ( 'NONE', #14799, 10.00000000000003197 ) ;
#7861=FACE_OUTER_BOUND ( 'NONE', #24700, .T. ) ;
#7866=DIRECTION ( 'NONE',  ( 0.000000000000000000, -1.132880637372608986E-16, 1.000000000000000000 ) ) ;
#7875=EDGE_CURVE ( 'NONE', #24589, #25420, #28582, .T. ) ;
#7878=FACE_OUTER_BOUND ( 'NONE', #15539, .T. ) ;
#7879=CIRCLE ( 'NONE', #25798, 0.7500000000000006661 ) ;
#7882=CIRCLE ( 'NONE', #13362, 0.7500000000000006661 ) ;
#7890=LINE ( 'NONE', #543, #24136 ) ;
#7905=CARTESIAN_POINT ( 'NONE',  ( 8.303920738747214259, 3.683253992019856149, -1.500000000000001332 ) ) ;
#7906=VECTOR ( 'NONE', #30468, 1000.000000000000000 ) ;
#7918=VERTEX_POINT ( 'NONE', #3813 ) ;
#7927=EDGE_CURVE ( 'NONE', #28059, #10427, #2687, .T. ) ;
#7941=DIRECTION ( 'NONE',  ( 0.000000000000000000, 1.000000000000000000, 1.193512090021232842E-16 ) ) ;
#7953=CARTESIAN_POINT ( 'NONE',  ( 9.184850993605159777E-16, -7.500000000000007994, -87.50000000000000000 ) ) ;
#7959=ORIENTED_EDGE ( 'NONE', *, *, #789, .F. ) ;
#7966=DIRECTION ( 'NONE',  ( 0.000000000000000000, -1.132880637372608986E-16, 1.000000000000000000 ) ) ;
#7982=AXIS2_PLACEMENT_3D ( 'NONE', #26280, #24088, #21906 ) ;
#7994=CIRCLE ( 'NONE', #18942, 0.7500000000000006661 ) ;
#8007=ORIENTED_EDGE ( 'NONE', *, *, #24456, .T. ) ;
#8010=DIRECTION ( 'NONE',  ( -0.000000000000000000, 1.132880637372608986E-16, -1.000000000000000000 ) ) ;
#8012=ORIENTED_EDGE ( 'NONE', *, *, #24279, .T. ) ;
#8015=AXIS2_PLACEMENT_3D ( 'NONE', #1860, #30543, #9040 ) ;
#8057=DIRECTION ( 'NONE',  ( 1.000000000000000000, 0.000000000000000000, -0.000000000000000000 ) ) ;
#8062=CARTESIAN_POINT ( 'NONE',  ( -7.730328572437709767, 4.608906612435681005, -1.500000000000001332 ) ) ;
#8066=CARTESIAN_POINT ( 'NONE',  ( 5.881244434206234217, 6.812559277181991391, 21.50000000000000000 ) ) ;
#8069=ADVANCED_FACE ( 'NONE', ( #6918 ), #4261, .F. ) ;
#8074=EDGE_CURVE ( 'NONE', #21028, #18115, #23285, .T. ) ;
#8098=EDGE_CURVE ( 'NONE', #1458, #20151, #25039, .T. ) ;
#8106=DIRECTION ( 'NONE',  ( 0.000000000000000000, 0.000000000000000000, 1.000000000000000000 ) ) ;
#8113=CIRCLE ( 'NONE', #610, 0.7499999999999997780 ) ;
#8116=DIRECTION ( 'NONE',  ( 1.000000000000000000, 0.000000000000000000, 0.000000000000000000 ) ) ;
#8118=LINE ( 'NONE', #27141, #14902 ) ;
#8132=AXIS2_PLACEMENT_3D ( 'NONE', #18275, #5805, #27799 ) ;
#8151=DIRECTION ( 'NONE',  ( 1.000000000000000000, 0.000000000000000000, 0.000000000000000000 ) ) ;
#8183=ORIENTED_EDGE ( 'NONE', *, *, #10090, .F. ) ;
#8194=DIRECTION ( 'NONE',  ( -0.000000000000000000, 1.132880637372608986E-16, -1.000000000000000000 ) ) ;
#8205=APPLICATION_CONTEXT ( 'automotive_design' ) ;
#8209=CARTESIAN_POINT ( 'NONE',  ( 1.530808498934191521E-15, -12.50000000000000000, -87.50000000000000000 ) ) ;
#8213=DIRECTION ( 'NONE',  ( 1.000000000000000000, 0.000000000000000000, 0.000000000000000000 ) ) ;
#8214=DIRECTION ( 'NONE',  ( 0.000000000000000000, 0.000000000000000000, 1.000000000000000000 ) ) ;
#8221=EDGE_CURVE ( 'NONE', #19990, #26044, #29050, .T. ) ;
#8222=DIRECTION ( 'NONE',  ( 1.000000000000000000, 0.000000000000000000, -0.000000000000000000 ) ) ;
#8229=VERTEX_POINT ( 'NONE', #26710 ) ;
#8241=EDGE_CURVE ( 'NONE', #9598, #9741, #657, .T. ) ;
#8244=DIRECTION ( 'NONE',  ( 0.000000000000000000, -1.132880637372608986E-16, 1.000000000000000000 ) ) ;
#8252=ORIENTED_EDGE ( 'NONE', *, *, #14683, .F. ) ;
#8262=CARTESIAN_POINT ( 'NONE',  ( 3.196529495465388226, 8.413215745755008967, -1.500000000000000888 ) ) ;
#8280=ORIENTED_EDGE ( 'NONE', *, *, #10532, .F. ) ;
#8287=AXIS2_PLACEMENT_3D ( 'NONE', #14814, #16857, #19348 ) ;
#8298=ORIENTED_EDGE ( 'NONE', *, *, #7473, .T. ) ;
#8310=VECTOR ( 'NONE', #1192, 1000.000000000000000 ) ;
#8311=EDGE_CURVE ( 'NONE', #19687, #30853, #8563, .T. ) ;
#8316=ORIENTED_EDGE ( 'NONE', *, *, #19851, .T. ) ;
#8343=ORIENTED_EDGE ( 'NONE', *, *, #22945, .T. ) ;
#8358=CARTESIAN_POINT ( 'NONE',  ( -5.687793815610304726, 6.974883619896852238, -3.621320343559650379 ) ) ;
#8362=AXIS2_PLACEMENT_3D ( 'NONE', #1717, #29818, #8460 ) ;
#8373=CIRCLE ( 'NONE', #25801, 9.084132297865673777 ) ;
#8385=PLANE ( 'NONE',  #12399 ) ;
#8391=DIRECTION ( 'NONE',  ( 1.000000000000000000, 0.000000000000000000, 0.000000000000000000 ) ) ;
#8393=ORIENTED_EDGE ( 'NONE', *, *, #14265, .F. ) ;
#8396=LINE ( 'NONE', #5586, #20726 ) ;
#8406=CARTESIAN_POINT ( 'NONE',  ( 3.763133143576435913, -8.268028093133381162, 21.50000000000000000 ) ) ;
#8411=CIRCLE ( 'NONE', #23332, 9.084132297865673777 ) ;
#8414=CARTESIAN_POINT ( 'NONE',  ( -1.438332125858111432, 8.884323311075791096, -1.500000000000000888 ) ) ;
#8420=CIRCLE ( 'NONE', #22388, 0.7500000000000006661 ) ;
#8432=CARTESIAN_POINT ( 'NONE',  ( 5.141690706682880752, -7.488956955540417404, 13.22130136205108819 ) ) ;
#8439=DIRECTION ( 'NONE',  ( 1.000000000000000000, 0.000000000000000000, 0.000000000000000000 ) ) ;
#8440=CIRCLE ( 'NONE', #18889, 0.7500000000000000000 ) ;
#8444=VERTEX_POINT ( 'NONE', #14792 ) ;
#8447=EDGE_CURVE ( 'NONE', #17647, #1314, #24999, .T. ) ;
#8460=DIRECTION ( 'NONE',  ( 1.000000000000000000, 0.000000000000000000, 0.000000000000000000 ) ) ;
#8467=VERTEX_POINT ( 'NONE', #25549 ) ;
#8475=CIRCLE ( 'NONE', #22405, 0.7500000000000002220 ) ;
#8478=LINE ( 'NONE', #22019, #454 ) ;
#8485=ORIENTED_EDGE ( 'NONE', *, *, #14321, .T. ) ;
#8487=ADVANCED_FACE ( 'NONE', ( #27741 ), #20247, .T. ) ;
#8489=LINE ( 'NONE', #24847, #1578 ) ;
#8492=CYLINDRICAL_SURFACE ( 'NONE', #19753, 0.7500000000000006661 ) ;
#8497=DIRECTION ( 'NONE',  ( -0.000000000000000000, 1.132880637372608986E-16, -1.000000000000000000 ) ) ;
#8503=ADVANCED_FACE ( 'NONE', ( #15718 ), #20551, .F. ) ;
#8504=AXIS2_PLACEMENT_3D ( 'NONE', #23161, #16464, #18509 ) ;
#8513=DIRECTION ( 'NONE',  ( 0.000000000000000000, 1.000000000000000000, 0.000000000000000000 ) ) ;
#8517=ORIENTED_EDGE ( 'NONE', *, *, #26947, .F. ) ;
#8523=CYLINDRICAL_SURFACE ( 'NONE', #371, 0.7500000000000006661 ) ;
#8525=ORIENTED_EDGE ( 'NONE', *, *, #24096, .F. ) ;
#8529=CARTESIAN_POINT ( 'NONE',  ( 0.000000000000000000, 1.699320956058915452E-16, -1.500000000000001776 ) ) ;
#8536=DIRECTION ( 'NONE',  ( 1.000000000000000000, 0.000000000000000000, 0.000000000000000000 ) ) ;
#8537=AXIS2_PLACEMENT_3D ( 'NONE', #17511, #29369, #6109 ) ;
#8541=VERTEX_POINT ( 'NONE', #3728 ) ;
#8543=DIRECTION ( 'NONE',  ( 0.000000000000000000, 1.132880637372608986E-16, -1.000000000000000000 ) ) ;
#8556=ORIENTED_EDGE ( 'NONE', *, *, #13204, .T. ) ;
#8563=CIRCLE ( 'NONE', #29976, 9.084132297865673777 ) ;
#8573=AXIS2_PLACEMENT_3D ( 'NONE', #4596, #23459, #8985 ) ;
#8593=ORIENTED_EDGE ( 'NONE', *, *, #24439, .F. ) ;
#8598=ORIENTED_EDGE ( 'NONE', *, *, #1927, .T. ) ;
#8627=EDGE_LOOP ( 'NONE', ( #18060, #19920, #4428, #23172 ) ) ;
#8643=DIRECTION ( 'NONE',  ( 0.000000000000000000, 0.000000000000000000, 1.000000000000000000 ) ) ;
#8662=ORIENTED_EDGE ( 'NONE', *, *, #17175, .F. ) ;
#8668=CIRCLE ( 'NONE', #9143, 0.7500000000000006661 ) ;
#8681=DIRECTION ( 'NONE',  ( 0.000000000000000000, 1.000000000000000000, 0.000000000000000000 ) ) ;
#8683=CARTESIAN_POINT ( 'NONE',  ( -6.062559277181930106, 5.881244434206302607, 21.50000000000000000 ) ) ;
#8684=DIRECTION ( 'NONE',  ( 0.000000000000000000, 0.000000000000000000, 1.000000000000000000 ) ) ;
#8691=LINE ( 'NONE', #29743, #5423 ) ;
#8697=DIRECTION ( 'NONE',  ( 0.000000000000000000, 1.000000000000000000, 1.193512090021232842E-16 ) ) ;
#8712=DIRECTION ( 'NONE',  ( 0.000000000000000000, 1.000000000000000000, 1.193512090021232842E-16 ) ) ;
#8717=ORIENTED_EDGE ( 'NONE', *, *, #15315, .T. ) ;
#8727=EDGE_LOOP ( 'NONE', ( #9644, #5607, #9650 ) ) ;
#8728=LINE ( 'NONE', #4191, #3807 ) ;
#8729=CARTESIAN_POINT ( 'NONE',  ( 0.000000000000000000, 10.00000000000003375, -87.50000000000000000 ) ) ;
#8732=CARTESIAN_POINT ( 'NONE',  ( 0.000000000000000000, 15.00000000000001954, 29.43090101791767665 ) ) ;
#8751=CARTESIAN_POINT ( 'NONE',  ( 8.197313248159948884, -3.914781618004724795, -1.500000000000002220 ) ) ;
#8755=LINE ( 'NONE', #13299, #27368 ) ;
#8762=LINE ( 'NONE', #545, #13316 ) ;
#8770=DIRECTION ( 'NONE',  ( -0.000000000000000000, 1.132880637372608986E-16, -1.000000000000000000 ) ) ;
#8772=CYLINDRICAL_SURFACE ( 'NONE', #14784, 0.7500000000000006661 ) ;
#8773=CARTESIAN_POINT ( 'NONE',  ( 2.516121109503181685, 8.728722367416592576, -1.500000000000000666 ) ) ;
#8777=DIRECTION ( 'NONE',  ( 0.000000000000000000, -1.132880637372608986E-16, 1.000000000000000000 ) ) ;
#8784=AXIS2_PLACEMENT_3D ( 'NONE', #13317, #25151, #29854 ) ;
#8800=AXIS2_PLACEMENT_3D ( 'NONE', #23422, #20632, #13325 ) ;
#8806=CIRCLE ( 'NONE', #3902, 0.7500000000000011102 ) ;
#8813=CARTESIAN_POINT ( 'NONE',  ( -6.974883619896829146, -5.687793815610328707, -1.500000000000002220 ) ) ;
#8834=CARTESIAN_POINT ( 'NONE',  ( -7.749586724479453181, -2.959227181723774525, -1.500000000000002220 ) ) ;
#8839=ORIENTED_EDGE ( 'NONE', *, *, #4616, .F. ) ;
#8845=AXIS2_PLACEMENT_3D ( 'NONE', #1220, #10720, #27724 ) ;
#8863=FACE_OUTER_BOUND ( 'NONE', #17465, .T. ) ;
#8864=DIRECTION ( 'NONE',  ( -0.000000000000000000, 1.132880637372608986E-16, -1.000000000000000000 ) ) ;
#8871=FACE_OUTER_BOUND ( 'NONE', #16013, .T. ) ;
#8880=ORIENTED_EDGE ( 'NONE', *, *, #24663, .F. ) ;
#8888=DIRECTION ( 'NONE',  ( 0.000000000000000000, 0.000000000000000000, 1.000000000000000000 ) ) ;
#8911=EDGE_CURVE ( 'NONE', #28030, #20761, #2880, .T. ) ;
#8923=VECTOR ( 'NONE', #15444, 1000.000000000000000 ) ;
#8925=CIRCLE ( 'NONE', #25836, 0.7500000000000006661 ) ;
#8930=AXIS2_PLACEMENT_3D ( 'NONE', #12917, #22704, #25206 ) ;
#8940=DIRECTION ( 'NONE',  ( -0.000000000000000000, -0.000000000000000000, 1.000000000000000000 ) ) ;
#8967=ORIENTED_EDGE ( 'NONE', *, *, #17426, .F. ) ;
#8968=AXIS2_PLACEMENT_3D ( 'NONE', #20268, #8888, #1699 ) ;
#8972=LINE ( 'NONE', #20808, #19337 ) ;
#8984=CARTESIAN_POINT ( 'NONE',  ( 0.000000000000000000, 12.50000000000000000, -87.50000000000000000 ) ) ;
#8985=DIRECTION ( 'NONE',  ( 0.000000000000000000, 1.000000000000000000, 0.000000000000000000 ) ) ;
#8991=CARTESIAN_POINT ( 'NONE',  ( -3.763133143576374628, 8.268028093133407808, 13.22130136205108997 ) ) ;
#9001=EDGE_CURVE ( 'NONE', #9137, #9666, #15275, .T. ) ;
#9002=FACE_OUTER_BOUND ( 'NONE', #7173, .T. ) ;
#9010=DIRECTION ( 'NONE',  ( 0.000000000000000000, 1.132880637372608986E-16, -1.000000000000000000 ) ) ;
#9014=DIRECTION ( 'NONE',  ( 1.000000000000000000, 0.000000000000000000, 0.000000000000000000 ) ) ;
#9022=DIRECTION ( 'NONE',  ( 0.000000000000000000, 1.000000000000000000, 0.000000000000000000 ) ) ;
#9024=LINE ( 'NONE', #16036, #21339 ) ;
#9030=VERTEX_POINT ( 'NONE', #12198 ) ;
#9036=CIRCLE ( 'NONE', #13021, 0.7500000000000002220 ) ;
#9037=DIRECTION ( 'NONE',  ( 0.000000000000000000, 1.000000000000000000, 1.193512090021232842E-16 ) ) ;
#9040=DIRECTION ( 'NONE',  ( 0.000000000000000000, 1.000000000000000000, 1.193512090021232842E-16 ) ) ;
#9043=EDGE_CURVE ( 'NONE', #21028, #1458, #1333, .T. ) ;
#9046=ORIENTED_EDGE ( 'NONE', *, *, #6512, .F. ) ;
#9056=LINE ( 'NONE', #16841, #21203 ) ;
#9071=VECTOR ( 'NONE', #21301, 1000.000000000000000 ) ;
#9076=CARTESIAN_POINT ( 'NONE',  ( -0.1262659238204836554, -8.999114229549588728, -3.621320343559650379 ) ) ;
#9081=EDGE_LOOP ( 'NONE', ( #8593, #16506 ) ) ;
#9092=CARTESIAN_POINT ( 'NONE',  ( -0.1262659238204836554, -8.999114229549588728, 21.50000000000000000 ) ) ;
#9097=DIRECTION ( 'NONE',  ( -0.000000000000000000, 1.132880637372608986E-16, -1.000000000000000000 ) ) ;
#9109=CARTESIAN_POINT ( 'NONE',  ( 0.000000000000000000, -2.435693370351110282E-15, 21.50000000000000355 ) ) ;
#9127=FACE_OUTER_BOUND ( 'NONE', #6994, .T. ) ;
#9137=VERTEX_POINT ( 'NONE', #5798 ) ;
#9141=DIRECTION ( 'NONE',  ( 1.000000000000000000, 0.000000000000000000, 0.000000000000000000 ) ) ;
#9143=AXIS2_PLACEMENT_3D ( 'NONE', #29157, #12948, #27135 ) ;
#9145=AXIS2_PLACEMENT_3D ( 'NONE', #30428, #30720, #2336 ) ;
#9150=EDGE_CURVE ( 'NONE', #18592, #6758, #3297, .T. ) ;
#9171=DIRECTION ( 'NONE',  ( 0.000000000000000000, 0.000000000000000000, 1.000000000000000000 ) ) ;
#9172=ORIENTED_EDGE ( 'NONE', *, *, #22538, .F. ) ;
#9176=ORIENTED_EDGE ( 'NONE', *, *, #25564, .F. ) ;
#9184=ORIENTED_EDGE ( 'NONE', *, *, #30735, .T. ) ;
#9185=LINE ( 'NONE', #14160, #28755 ) ;
#9198=CARTESIAN_POINT ( 'NONE',  ( 0.000000000000000000, 1.699320956058915452E-16, -1.500000000000001776 ) ) ;
#9210=CARTESIAN_POINT ( 'NONE',  ( -5.141690706682822132, 7.488956955540452931, 13.22130136205108819 ) ) ;
#9231=FACE_OUTER_BOUND ( 'NONE', #8727, .T. ) ;
#9242=CYLINDRICAL_SURFACE ( 'NONE', #19522, 0.7500000000000006661 ) ;
#9251=CIRCLE ( 'NONE', #18232, 9.084132297865673777 ) ;
#9274=VERTEX_POINT ( 'NONE', #22787 ) ;
#9283=AXIS2_PLACEMENT_3D ( 'NONE', #26467, #10230, #2455 ) ;
#9285=VERTEX_POINT ( 'NONE', #22937 ) ;
#9289=DIRECTION ( 'NONE',  ( 0.000000000000000000, -1.132880637372608986E-16, 1.000000000000000000 ) ) ;
#9302=PLANE ( 'NONE',  #13559 ) ;
#9310=CARTESIAN_POINT ( 'NONE',  ( 0.1262659238204208167, 8.999114229549594057, -3.621320343559650379 ) ) ;
#9312=AXIS2_PLACEMENT_3D ( 'NONE', #20611, #22223, #22386 ) ;
#9317=CARTESIAN_POINT ( 'NONE',  ( -8.999114229549592281, 0.1262659238205133538, -3.621320343559650379 ) ) ;
#9334=DIRECTION ( 'NONE',  ( 0.000000000000000000, 0.000000000000000000, 1.000000000000000000 ) ) ;
#9348=AXIS2_PLACEMENT_3D ( 'NONE', #23390, #1723, #25736 ) ;
#9361=ORIENTED_EDGE ( 'NONE', *, *, #29930, .T. ) ;
#9362=CIRCLE ( 'NONE', #23722, 0.7500000000000006661 ) ;
#9363=DIRECTION ( 'NONE',  ( 1.000000000000000000, 0.000000000000000000, -0.000000000000000000 ) ) ;
#9397=EDGE_CURVE ( 'NONE', #6758, #17047, #24282, .T. ) ;
#9415=CARTESIAN_POINT ( 'NONE',  ( -7.663215745754974328, 3.196529495465474380, -3.621320343559650379 ) ) ;
#9418=CARTESIAN_POINT ( 'NONE',  ( -5.687793815610304726, 6.974883619896852238, -3.621320343559650379 ) ) ;
#9419=ORIENTED_EDGE ( 'NONE', *, *, #17393, .F. ) ;
#9422=DIRECTION ( 'NONE',  ( -0.000000000000000000, 1.132880637372608986E-16, -1.000000000000000000 ) ) ;
#9437=CARTESIAN_POINT ( 'NONE',  ( 1.224646799147357990E-15, -10.00000000000006395, 157.4999999999999716 ) ) ;
#9440=ORIENTED_EDGE ( 'NONE', *, *, #9575, .F. ) ;
#9450=VERTEX_POINT ( 'NONE', #15250 ) ;
#9461=VERTEX_POINT ( 'NONE', #1084 ) ;
#9479=DIRECTION ( 'NONE',  ( 1.000000000000000000, 0.000000000000000000, 0.000000000000000000 ) ) ;
#9482=CARTESIAN_POINT ( 'NONE',  ( 8.159193615868399974, -3.993622308618911099, 13.22130136205108819 ) ) ;
#9486=CARTESIAN_POINT ( 'NONE',  ( 0.000000000000000000, 0.000000000000000000, 0.000000000000000000 ) ) ;
#9490=EDGE_LOOP ( 'NONE', ( #3561, #355, #20410, #19809 ) ) ;
#9503=LINE ( 'NONE', #28534, #10852 ) ;
#9508=DIRECTION ( 'NONE',  ( -0.000000000000000000, 1.132880637372608986E-16, -1.000000000000000000 ) ) ;
#9515=CARTESIAN_POINT ( 'NONE',  ( 5.687793815610356241, -6.974883619896809606, 21.50000000000000000 ) ) ;
#9523=CARTESIAN_POINT ( 'NONE',  ( -0.1262659238204836554, -8.999114229549588728, 21.50000000000000000 ) ) ;
#9534=EDGE_CURVE ( 'NONE', #30279, #25497, #29769, .T. ) ;
#9537=CYLINDRICAL_SURFACE ( 'NONE', #6334, 9.084132297865673777 ) ;
#9551=DIRECTION ( 'NONE',  ( 0.000000000000000000, 0.000000000000000000, 1.000000000000000000 ) ) ;
#9559=ORIENTED_EDGE ( 'NONE', *, *, #22685, .F. ) ;
#9560=LINE ( 'NONE', #4263, #25072 ) ;
#9575=EDGE_CURVE ( 'NONE', #28301, #29154, #22764, .T. ) ;
#9578=CARTESIAN_POINT ( 'NONE',  ( -5.881244434206279514, -6.812559277181949646, 21.50000000000000000 ) ) ;
#9587=EDGE_LOOP ( 'NONE', ( #13873, #19029, #14727, #5676 ) ) ;
#9598=VERTEX_POINT ( 'NONE', #29939 ) ;
#9606=PRODUCT_CONTEXT ( 'NONE', #26509, 'mechanical' ) ;
#9644=ORIENTED_EDGE ( 'NONE', *, *, #20586, .F. ) ;
#9650=ORIENTED_EDGE ( 'NONE', *, *, #20841, .F. ) ;
#9666=VERTEX_POINT ( 'NONE', #5406 ) ;
#9672=DIRECTION ( 'NONE',  ( 0.000000000000000000, 1.000000000000000000, 0.000000000000000000 ) ) ;
#9687=CARTESIAN_POINT ( 'NONE',  ( -1.438332125858111432, 8.884323311075791096, 21.50000000000000000 ) ) ;
#9689=CIRCLE ( 'NONE', #27140, 0.7500000000000006661 ) ;
#9697=ADVANCED_FACE ( 'NONE', ( #19737 ), #24893, .F. ) ;
#9710=EDGE_LOOP ( 'NONE', ( #23807, #18422, #23240, #19469 ) ) ;
#9720=CARTESIAN_POINT ( 'NONE',  ( 0.000000000000000000, 9.084132297865672001, 21.50000000000000355 ) ) ;
#9740=CARTESIAN_POINT ( 'NONE',  ( 0.000000000000000000, -8.043452525345523162E-15, -16.50000000000000000 ) ) ;
#9741=VERTEX_POINT ( 'NONE', #1032 ) ;
#9747=DIRECTION ( 'NONE',  ( 0.000000000000000000, 0.000000000000000000, 1.000000000000000000 ) ) ;
#9761=DIRECTION ( 'NONE',  ( 0.000000000000000000, 1.132880637372608986E-16, -1.000000000000000000 ) ) ;
#9777=CARTESIAN_POINT ( 'NONE',  ( 0.000000000000000000, -1.307826893540337417E-14, 27.94260272410217638 ) ) ;
#9780=EDGE_CURVE ( 'NONE', #11004, #191, #20810, .T. ) ;
#9791=ORIENTED_EDGE ( 'NONE', *, *, #15663, .F. ) ;
#9792=AXIS2_PLACEMENT_3D ( 'NONE', #21248, #27572, #30778 ) ;
#9795=EDGE_CURVE ( 'NONE', #11295, #11064, #16293, .T. ) ;
#9800=CARTESIAN_POINT ( 'NONE',  ( 7.392982946727082449, -5.278755796068694828, 13.22130136205108819 ) ) ;
#9823=ORIENTED_EDGE ( 'NONE', *, *, #16067, .F. ) ;
#9832=ORIENTED_EDGE ( 'NONE', *, *, #13347, .F. ) ;
#9835=DIRECTION ( 'NONE',  ( 1.000000000000000000, 0.000000000000000000, 0.000000000000000000 ) ) ;
#9841=AXIS2_PLACEMENT_3D ( 'NONE', #16211, #18710, #6851 ) ;
#9843=DIRECTION ( 'NONE',  ( 0.000000000000000000, 0.000000000000000000, 1.000000000000000000 ) ) ;
#9851=CIRCLE ( 'NONE', #13342, 9.084132297865673777 ) ;
#9858=CARTESIAN_POINT ( 'NONE',  ( -8.249114229549590505, 0.1262659238205133538, -3.621320343559650379 ) ) ;
#9863=DIRECTION ( 'NONE',  ( 1.000000000000000000, 0.000000000000000000, 0.000000000000000000 ) ) ;
#9867=DIRECTION ( 'NONE',  ( 1.000000000000000000, 0.000000000000000000, 0.000000000000000000 ) ) ;
#9872=VERTEX_POINT ( 'NONE', #28608 ) ;
#9879=ORIENTED_EDGE ( 'NONE', *, *, #20040, .F. ) ;
#9883=AXIS2_PLACEMENT_3D ( 'NONE', #12272, #28650, #411 ) ;
#9910=CARTESIAN_POINT ( 'NONE',  ( 0.000000000000000000, -2.435693370351110282E-15, 21.50000000000000355 ) ) ;
#9914=ORIENTED_EDGE ( 'NONE', *, *, #27287, .T. ) ;
#9929=ADVANCED_FACE ( 'NONE', ( #7861 ), #21891, .F. ) ;
#9930=DIRECTION ( 'NONE',  ( 1.000000000000000000, 0.000000000000000000, 0.000000000000000000 ) ) ;
#9938=FACE_BOUND ( 'NONE', #20612, .T. ) ;
#9939=ORIENTED_EDGE ( 'NONE', *, *, #28839, .F. ) ;
#9942=AXIS2_PLACEMENT_3D ( 'NONE', #15979, #30775, #3980 ) ;
#9948=DIRECTION ( 'NONE',  ( -0.000000000000000000, -0.000000000000000000, 1.000000000000000000 ) ) ;
#9962=EDGE_CURVE ( 'NONE', #16597, #17742, #15017, .T. ) ;
#9969=CARTESIAN_POINT ( 'NONE',  ( -7.856594496258223259, -4.390207617113929039, -1.500000000000002220 ) ) ;
#9977=CARTESIAN_POINT ( 'NONE',  ( 7.856594496258195726, 4.390207617113981442, 21.50000000000000000 ) ) ;
#9981=DIRECTION ( 'NONE',  ( -0.000000000000000000, 1.132880637372608986E-16, -1.000000000000000000 ) ) ;
#9984=VERTEX_POINT ( 'NONE', #8773 ) ;
#9989=AXIS2_PLACEMENT_3D ( 'NONE', #30730, #28873, #9835 ) ;
#9995=CARTESIAN_POINT ( 'NONE',  ( -1.687027447297492211, -8.840471615930066918, 21.50000000000000000 ) ) ;
#9999=ADVANCED_FACE ( 'NONE', ( #23108 ), #15959, .F. ) ;
#10000=ORIENTED_EDGE ( 'NONE', *, *, #22171, .T. ) ;
#10010=DIRECTION ( 'NONE',  ( -0.000000000000000000, 1.132880637372608986E-16, -1.000000000000000000 ) ) ;
#10018=ORIENTED_EDGE ( 'NONE', *, *, #26131, .T. ) ;
#10030=CARTESIAN_POINT ( 'NONE',  ( -2.959227181723746547, 8.499586724479465616, -1.500000000000000888 ) ) ;
#10032=CARTESIAN_POINT ( 'NONE',  ( -6.301234758012549619, 6.543385983536412098, 13.22130136205108819 ) ) ;
#10034=ORIENTED_EDGE ( 'NONE', *, *, #7655, .F. ) ;
#10041=DIRECTION ( 'NONE',  ( 1.000000000000000000, 0.000000000000000000, 0.000000000000000000 ) ) ;
#10049=ORIENTED_EDGE ( 'NONE', *, *, #7106, .T. ) ;
#10051=DIRECTION ( 'NONE',  ( 1.000000000000000000, 0.000000000000000000, 0.000000000000000000 ) ) ;
#10065=DIRECTION ( 'NONE',  ( -0.000000000000000000, -0.000000000000000000, 1.000000000000000000 ) ) ;
#10073=DIRECTION ( 'NONE',  ( 0.000000000000000000, 1.000000000000000000, 1.193512090021232842E-16 ) ) ;
#10077=DIRECTION ( 'NONE',  ( 0.000000000000000000, 1.000000000000000000, 0.000000000000000000 ) ) ;
#10083=CARTESIAN_POINT ( 'NONE',  ( -6.812559277181930106, 5.881244434206302607, 21.50000000000000000 ) ) ;
#10084=DIRECTION ( 'NONE',  ( 0.000000000000000000, 1.000000000000000000, 0.000000000000000000 ) ) ;
#10090=EDGE_CURVE ( 'NONE', #26641, #5849, #16749, .T. ) ;
#10103=CARTESIAN_POINT ( 'NONE',  ( 8.268028093133366951, 3.763133143576461670, 21.50000000000000000 ) ) ;
#10172=CARTESIAN_POINT ( 'NONE',  ( -2.185336383880142730, 8.817355867515834333, 13.22130136205108997 ) ) ;
#10199=CARTESIAN_POINT ( 'NONE',  ( -3.763133143576374628, 8.268028093133407808, -1.500000000000000888 ) ) ;
#10203=LINE ( 'NONE', #21438, #17399 ) ;
#10205=VERTEX_POINT ( 'NONE', #11363 ) ;
#10206=ORIENTED_EDGE ( 'NONE', *, *, #25564, .T. ) ;
#10212=VERTEX_POINT ( 'NONE', #18221 ) ;
#10230=DIRECTION ( 'NONE',  ( 0.000000000000000000, -1.132880637372608986E-16, 1.000000000000000000 ) ) ;
#10232=EDGE_CURVE ( 'NONE', #21461, #3179, #7320, .T. ) ;
#10254=AXIS2_PLACEMENT_3D ( 'NONE', #30020, #5850, #13498 ) ;
#10256=CARTESIAN_POINT ( 'NONE',  ( 0.000000000000000000, 1.699320956058915452E-16, -1.500000000000001776 ) ) ;
#10281=ORIENTED_EDGE ( 'NONE', *, *, #27310, .T. ) ;
#10308=LINE ( 'NONE', #27162, #8923 ) ;
#10309=CARTESIAN_POINT ( 'NONE',  ( 0.000000000000000000, -2.435693370351110282E-15, 21.50000000000000355 ) ) ;
#10322=DIRECTION ( 'NONE',  ( -0.000000000000000000, -0.000000000000000000, 1.000000000000000000 ) ) ;
#10325=EDGE_CURVE ( 'NONE', #1559, #25155, #4778, .T. ) ;
#10326=DIRECTION ( 'NONE',  ( 0.000000000000000000, 0.000000000000000000, 1.000000000000000000 ) ) ;
#10344=CARTESIAN_POINT ( 'NONE',  ( 2.959227181723801170, -8.499586724479446076, 21.50000000000000000 ) ) ;
#10358=ORIENTED_EDGE ( 'NONE', *, *, #24207, .F. ) ;
#10365=EDGE_CURVE ( 'NONE', #1662, #24166, #17760, .T. ) ;
#10367=DIRECTION ( 'NONE',  ( 1.000000000000000000, 0.000000000000000000, -0.000000000000000000 ) ) ;
#10369=ORIENTED_EDGE ( 'NONE', *, *, #5973, .F. ) ;
#10376=ORIENTED_EDGE ( 'NONE', *, *, #21027, .F. ) ;
#10380=EDGE_CURVE ( 'NONE', #16368, #9274, #21732, .T. ) ;
#10381=ORIENTED_EDGE ( 'NONE', *, *, #27045, .F. ) ;
#10410=AXIS2_PLACEMENT_3D ( 'NONE', #22944, #25295, #6263 ) ;
#10413=DIRECTION ( 'NONE',  ( 0.000000000000000000, -1.132880637372608986E-16, 1.000000000000000000 ) ) ;
#10417=ORIENTED_EDGE ( 'NONE', *, *, #1909, .F. ) ;
#10420=DIRECTION ( 'NONE',  ( 1.000000000000000000, 0.000000000000000000, 0.000000000000000000 ) ) ;
#10425=AXIS2_PLACEMENT_3D ( 'NONE', #1657, #25972, #4598 ) ;
#10427=VERTEX_POINT ( 'NONE', #24728 ) ;
#10429=DIRECTION ( 'NONE',  ( 0.000000000000000000, 1.000000000000000000, 0.000000000000000000 ) ) ;
#10460=CARTESIAN_POINT ( 'NONE',  ( 0.000000000000000000, 1.699320956058915452E-16, -1.500000000000001776 ) ) ;
#10483=VECTOR ( 'NONE', #2845, 1000.000000000000000 ) ;
#10490=CARTESIAN_POINT ( 'NONE',  ( -6.812559277181930106, 5.881244434206302607, -1.500000000000000888 ) ) ;
#10511=DIRECTION ( 'NONE',  ( 0.000000000000000000, 1.132880637372608986E-16, -1.000000000000000000 ) ) ;
#10515=AXIS2_PLACEMENT_3D ( 'NONE', #16035, #29617, #8712 ) ;
#10517=ORIENTED_EDGE ( 'NONE', *, *, #10380, .F. ) ;
#10518=ORIENTED_EDGE ( 'NONE', *, *, #28987, .T. ) ;
#10532=EDGE_CURVE ( 'NONE', #9285, #7702, #12589, .T. ) ;
#10551=CARTESIAN_POINT ( 'NONE',  ( 0.000000000000000000, 1.699320956058915452E-16, -1.500000000000001776 ) ) ;
#10552=DIRECTION ( 'NONE',  ( 0.000000000000000000, 0.000000000000000000, 1.000000000000000000 ) ) ;
#10553=VERTEX_POINT ( 'NONE', #30185 ) ;
#10559=CARTESIAN_POINT ( 'NONE',  ( 0.000000000000000000, -2.435693370351110282E-15, 21.50000000000000355 ) ) ;
#10563=ADVANCED_FACE ( 'NONE', ( #11619 ), #3835, .F. ) ;
#10565=AXIS2_PLACEMENT_3D ( 'NONE', #22721, #9843, #13234 ) ;
#10593=CARTESIAN_POINT ( 'NONE',  ( -8.728722367416567707, 2.516121109503271835, 13.22130136205108819 ) ) ;
#10606=ORIENTED_EDGE ( 'NONE', *, *, #17668, .F. ) ;
#10623=CARTESIAN_POINT ( 'NONE',  ( 3.683253992019827727, -8.303920738747228469, 21.50000000000000000 ) ) ;
#10645=ORIENTED_EDGE ( 'NONE', *, *, #26618, .F. ) ;
#10646=ORIENTED_EDGE ( 'NONE', *, *, #13979, .T. ) ;
#10664=EDGE_CURVE ( 'NONE', #29091, #19074, #4451, .T. ) ;
#10669=ORIENTED_EDGE ( 'NONE', *, *, #30510, .T. ) ;
#10700=DIRECTION ( 'NONE',  ( -0.000000000000000000, -0.000000000000000000, 1.000000000000000000 ) ) ;
#10720=DIRECTION ( 'NONE',  ( 0.000000000000000000, -1.132880637372608986E-16, 1.000000000000000000 ) ) ;
#10721=FACE_OUTER_BOUND ( 'NONE', #28657, .T. ) ;
#10724=CIRCLE ( 'NONE', #14698, 9.084132297865673777 ) ;
#10731=CARTESIAN_POINT ( 'NONE',  ( 5.141690706682880752, -7.488956955540417404, -1.500000000000002665 ) ) ;
#10758=DIRECTION ( 'NONE',  ( 0.000000000000000000, -1.132880637372608986E-16, 1.000000000000000000 ) ) ;
#10775=AXIS2_PLACEMENT_3D ( 'NONE', #16052, #9334, #15738 ) ;
#10786=ORIENTED_EDGE ( 'NONE', *, *, #11617, .F. ) ;
#10788=VECTOR ( 'NONE', #28897, 1000.000000000000000 ) ;
#10791=DIRECTION ( 'NONE',  ( 0.000000000000000000, 1.000000000000000000, 1.193512090021232842E-16 ) ) ;
#10793=DIRECTION ( 'NONE',  ( 1.000000000000000000, 0.000000000000000000, 0.000000000000000000 ) ) ;
#10817=AXIS2_PLACEMENT_3D ( 'NONE', #22810, #13153, #20616 ) ;
#10822=ORIENTED_EDGE ( 'NONE', *, *, #1232, .F. ) ;
#10835=CARTESIAN_POINT ( 'NONE',  ( -0.9370274472974918778, -8.840471615930066918, -3.621320343559650379 ) ) ;
#10845=AXIS2_PLACEMENT_3D ( 'NONE', #17448, #20401, #12930 ) ;
#10852=VECTOR ( 'NONE', #20775, 1000.000000000000000 ) ;
#10858=DIRECTION ( 'NONE',  ( 1.000000000000000000, 0.000000000000000000, 0.000000000000000000 ) ) ;
#10872=AXIS2_PLACEMENT_3D ( 'NONE', #24476, #12488, #21829 ) ;
#10902=EDGE_CURVE ( 'NONE', #17876, #897, #24820, .T. ) ;
#10903=AXIS2_PLACEMENT_3D ( 'NONE', #2288, #13855, #9479 ) ;
#10911=AXIS2_PLACEMENT_3D ( 'NONE', #30199, #9289, #13681 ) ;
#10916=DIRECTION ( 'NONE',  ( -0.000000000000000000, -0.000000000000000000, 1.000000000000000000 ) ) ;
#10925=EDGE_CURVE ( 'NONE', #1692, #17876, #20280, .T. ) ;
#10933=VERTEX_POINT ( 'NONE', #22008 ) ;
#10935=EDGE_CURVE ( 'NONE', #12072, #21461, #4283, .T. ) ;
#10936=EDGE_LOOP ( 'NONE', ( #89, #21873, #22262, #20907, #13417 ) ) ;
#10937=AXIS2_PLACEMENT_3D ( 'NONE', #472, #2809, #4834 ) ;
#10959=VECTOR ( 'NONE', #1410, 1000.000000000000000 ) ;
#10960=DIRECTION ( 'NONE',  ( 1.000000000000000000, 0.000000000000000000, 0.000000000000000000 ) ) ;
#10984=DIRECTION ( 'NONE',  ( 0.000000000000000000, 0.000000000000000000, 1.000000000000000000 ) ) ;
#10987=CARTESIAN_POINT ( 'NONE',  ( 1.438332125858173605, -8.884323311075778662, 21.50000000000000000 ) ) ;
#10991=ORIENTED_EDGE ( 'NONE', *, *, #7295, .T. ) ;
#11001=VERTEX_POINT ( 'NONE', #18263 ) ;
#11002=DIRECTION ( 'NONE',  ( -0.000000000000000000, -0.000000000000000000, 1.000000000000000000 ) ) ;
#11004=VERTEX_POINT ( 'NONE', #15605 ) ;
#11021=PLANE ( 'NONE',  #26023 ) ;
#11030=CARTESIAN_POINT ( 'NONE',  ( -7.730328572437709767, 4.608906612435681005, 21.50000000000000000 ) ) ;
#11032=ORIENTED_EDGE ( 'NONE', *, *, #11034, .F. ) ;
#11034=EDGE_CURVE ( 'NONE', #2118, #13370, #5787, .T. ) ;
#11038=DIRECTION ( 'NONE',  ( 0.000000000000000000, 1.000000000000000000, 0.000000000000000000 ) ) ;
#11046=VECTOR ( 'NONE', #808, 1000.000000000000000 ) ;
#11052=DIRECTION ( 'NONE',  ( 1.000000000000000000, 0.000000000000000000, 0.000000000000000000 ) ) ;
#11064=VERTEX_POINT ( 'NONE', #26354 ) ;
#11067=DIRECTION ( 'NONE',  ( 0.000000000000000000, 1.132880637372608986E-16, -1.000000000000000000 ) ) ;
#11077=CIRCLE ( 'NONE', #16536, 12.50000000000000000 ) ;
#11078=ORIENTED_EDGE ( 'NONE', *, *, #3805, .T. ) ;
#11084=EDGE_CURVE ( 'NONE', #11358, #12072, #23846, .T. ) ;
#11090=EDGE_LOOP ( 'NONE', ( #15043, #15963, #30291, #11429 ) ) ;
#11124=CARTESIAN_POINT ( 'NONE',  ( 5.349779314757592275, 7.341751895053254096, 21.50000000000000000 ) ) ;
#11131=ORIENTED_EDGE ( 'NONE', *, *, #24666, .F. ) ;
#11133=LINE ( 'NONE', #23117, #18821 ) ;
#11135=EDGE_CURVE ( 'NONE', #15425, #11338, #24177, .T. ) ;
#11152=VERTEX_POINT ( 'NONE', #28870 ) ;
#11163=ORIENTED_EDGE ( 'NONE', *, *, #1023, .F. ) ;
#11168=DIRECTION ( 'NONE',  ( 1.000000000000000000, 0.000000000000000000, 0.000000000000000000 ) ) ;
#11176=DIRECTION ( 'NONE',  ( 1.000000000000000000, 0.000000000000000000, 0.000000000000000000 ) ) ;
#11178=DIRECTION ( 'NONE',  ( 0.000000000000000000, -1.132880637372608986E-16, 1.000000000000000000 ) ) ;
#11184=ORIENTED_EDGE ( 'NONE', *, *, #4203, .F. ) ;
#11191=FACE_OUTER_BOUND ( 'NONE', #30514, .T. ) ;
#11192=FACE_OUTER_BOUND ( 'NONE', #29587, .T. ) ;
#11198=CARTESIAN_POINT ( 'NONE',  ( -8.413215745754975217, 3.196529495465474380, 21.50000000000000000 ) ) ;
#11213=CARTESIAN_POINT ( 'NONE',  ( -9.033033306777449312, 0.9621688436940325495, 21.50000000000000000 ) ) ;
#11214=CIRCLE ( 'NONE', #20161, 0.7500000000000015543 ) ;
#11220=ORIENTED_EDGE ( 'NONE', *, *, #22415, .T. ) ;
#11223=ORIENTED_EDGE ( 'NONE', *, *, #14318, .F. ) ;
#11244=DIRECTION ( 'NONE',  ( 1.000000000000000000, 0.000000000000000000, -0.000000000000000000 ) ) ;
#11258=EDGE_CURVE ( 'NONE', #11338, #5002, #7271, .T. ) ;
#11263=EDGE_CURVE ( 'NONE', #15560, #4711, #25709, .T. ) ;
#11265=CARTESIAN_POINT ( 'NONE',  ( 0.6237340761795171495, -8.999114229549588728, -3.621320343559650379 ) ) ;
#11266=EDGE_CURVE ( 'NONE', #27939, #24466, #783, .T. ) ;
#11267=DIRECTION ( 'NONE',  ( -0.000000000000000000, -0.000000000000000000, 1.000000000000000000 ) ) ;
#11292=LINE ( 'NONE', #9415, #3699 ) ;
#11295=VERTEX_POINT ( 'NONE', #13110 ) ;
#11302=ORIENTED_EDGE ( 'NONE', *, *, #28196, .T. ) ;
#11305=CIRCLE ( 'NONE', #24738, 9.084132297865673777 ) ;
#11309=AXIS2_PLACEMENT_3D ( 'NONE', #30140, #8770, #3638 ) ;
#11311=EDGE_CURVE ( 'NONE', #11004, #4539, #13260, .T. ) ;
#11313=CARTESIAN_POINT ( 'NONE',  ( -8.134323311075783991, -1.438332125858144295, 21.50000000000000000 ) ) ;
#11324=CARTESIAN_POINT ( 'NONE',  ( 0.000000000000000000, 1.604273173167211147E-31, -87.50000000000000000 ) ) ;
#11327=FACE_OUTER_BOUND ( 'NONE', #21766, .T. ) ;
#11330=AXIS2_PLACEMENT_3D ( 'NONE', #9076, #16394, #15950 ) ;
#11338=VERTEX_POINT ( 'NONE', #23053 ) ;
#11345=ORIENTED_EDGE ( 'NONE', *, *, #26947, .T. ) ;
#11352=DIRECTION ( 'NONE',  ( 1.000000000000000000, 0.000000000000000000, 0.000000000000000000 ) ) ;
#11355=DIRECTION ( 'NONE',  ( 0.000000000000000000, 1.000000000000000000, 1.193512090021232842E-16 ) ) ;
#11358=VERTEX_POINT ( 'NONE', #23371 ) ;
#11360=DIRECTION ( 'NONE',  ( -0.000000000000000000, -0.000000000000000000, 1.000000000000000000 ) ) ;
#11361=CYLINDRICAL_SURFACE ( 'NONE', #17208, 7.500000000000007994 ) ;
#11363=CARTESIAN_POINT ( 'NONE',  ( -7.488956955540436056, -5.141690706682852330, 21.50000000000000000 ) ) ;
#11364=FACE_OUTER_BOUND ( 'NONE', #11090, .T. ) ;
#11367=DIRECTION ( 'NONE',  ( 0.000000000000000000, 0.000000000000000000, 1.000000000000000000 ) ) ;
#11369=VECTOR ( 'NONE', #2500, 1000.000000000000000 ) ;
#11380=CIRCLE ( 'NONE', #18347, 9.084132297865673777 ) ;
#11382=VERTEX_POINT ( 'NONE', #30687 ) ;
#11392=CIRCLE ( 'NONE', #28820, 0.7500000000000006661 ) ;
#11425=ORIENTED_EDGE ( 'NONE', *, *, #6869, .F. ) ;
#11426=CARTESIAN_POINT ( 'NONE',  ( 4.608906612435600181, 7.730328572437758616, -1.500000000000000888 ) ) ;
#11427=CIRCLE ( 'NONE', #17909, 0.7500000000000001110 ) ;
#11428=DIRECTION ( 'NONE',  ( -0.000000000000000000, -0.000000000000000000, 1.000000000000000000 ) ) ;
#11429=ORIENTED_EDGE ( 'NONE', *, *, #5452, .F. ) ;
#11430=LINE ( 'NONE', #11265, #26787 ) ;
#11436=DIRECTION ( 'NONE',  ( -0.000000000000000000, 1.132880637372608986E-16, -1.000000000000000000 ) ) ;
#11439=DIRECTION ( 'NONE',  ( 1.000000000000000000, 0.000000000000000000, 0.000000000000000000 ) ) ;
#11441=ADVANCED_FACE ( 'NONE', ( #13428 ), #30093, .F. ) ;
#11453=DIRECTION ( 'NONE',  ( -0.000000000000000000, -0.000000000000000000, 1.000000000000000000 ) ) ;
#11456=ORIENTED_EDGE ( 'NONE', *, *, #1825, .F. ) ;
#11459=VERTEX_POINT ( 'NONE', #25570 ) ;
#11460=EDGE_CURVE ( 'NONE', #28009, #7211, #8728, .T. ) ;
#11479=CARTESIAN_POINT ( 'NONE',  ( -4.390207617113899730, 7.856594496258241023, 21.50000000000000000 ) ) ;
#11483=AXIS2_PLACEMENT_3D ( 'NONE', #9523, #16860, #5000 ) ;
#11505=CARTESIAN_POINT ( 'NONE',  ( 0.000000000000000000, 1.699320956058915452E-16, -1.500000000000001776 ) ) ;
#11506=VECTOR ( 'NONE', #14632, 1000.000000000000000 ) ;
#11508=ORIENTED_EDGE ( 'NONE', *, *, #21388, .T. ) ;
#11511=CIRCLE ( 'NONE', #8537, 0.7500000000000006661 ) ;
#11519=VERTEX_POINT ( 'NONE', #12757 ) ;
#11529=EDGE_LOOP ( 'NONE', ( #16900, #6462, #22742, #18849 ) ) ;
#11541=EDGE_LOOP ( 'NONE', ( #25589, #1082, #15476, #1380 ) ) ;
#11549=VERTEX_POINT ( 'NONE', #20082 ) ;
#11560=CYLINDRICAL_SURFACE ( 'NONE', #20856, 0.7500000000000011102 ) ;
#11562=VERTEX_POINT ( 'NONE', #3553 ) ;
#11577=EDGE_CURVE ( 'NONE', #24166, #20151, #8396, .T. ) ;
#11583=DIRECTION ( 'NONE',  ( 0.000000000000000000, 1.132880637372608986E-16, -1.000000000000000000 ) ) ;
#11585=FACE_OUTER_BOUND ( 'NONE', #28013, .T. ) ;
#11589=DIRECTION ( 'NONE',  ( 0.000000000000000000, 1.000000000000000000, 0.000000000000000000 ) ) ;
#11590=AXIS2_PLACEMENT_3D ( 'NONE', #28903, #14550, #24047 ) ;
#11591=CIRCLE ( 'NONE', #29025, 9.084132297865673777 ) ;
#11592=DIRECTION ( 'NONE',  ( 0.000000000000000000, -1.132880637372608986E-16, 1.000000000000000000 ) ) ;
#11597=DIRECTION ( 'NONE',  ( 0.000000000000000000, 1.000000000000000000, 1.193512090021232842E-16 ) ) ;
#11602=DIRECTION ( 'NONE',  ( -0.000000000000000000, -0.000000000000000000, 1.000000000000000000 ) ) ;
#11614=CARTESIAN_POINT ( 'NONE',  ( 1.112485354161228759E-15, -9.084132297865675554, 21.50000000000000355 ) ) ;
#11617=EDGE_CURVE ( 'NONE', #14972, #18098, #20536, .T. ) ;
#11619=FACE_OUTER_BOUND ( 'NONE', #12958, .T. ) ;
#11645=EDGE_CURVE ( 'NONE', #17647, #10553, #25218, .T. ) ;
#11653=PRODUCT_DEFINITION_SHAPE ( 'NONE', 'NONE',  #22874 ) ;
#11659=CARTESIAN_POINT ( 'NONE',  ( -3.196529495465446402, -8.413215745754985875, 21.50000000000000000 ) ) ;
#11663=CARTESIAN_POINT ( 'NONE',  ( -0.1262659238204836554, -8.999114229549588728, 21.50000000000000000 ) ) ;
#11664=EDGE_CURVE ( 'NONE', #9274, #7713, #20255, .T. ) ;
#11684=VERTEX_POINT ( 'NONE', #18055 ) ;
#11686=ADVANCED_FACE ( 'NONE', ( #4889 ), #11754, .F. ) ;
#11695=CARTESIAN_POINT ( 'NONE',  ( -0.6883321258581104329, 8.884323311075791096, -1.500000000000000888 ) ) ;
#11699=ORIENTED_EDGE ( 'NONE', *, *, #25240, .F. ) ;
#11721=AXIS2_PLACEMENT_3D ( 'NONE', #9995, #19500, #4305 ) ;
#11722=DIRECTION ( 'NONE',  ( 0.000000000000000000, 0.000000000000000000, 1.000000000000000000 ) ) ;
#11724=DIRECTION ( 'NONE',  ( 1.000000000000000000, 0.000000000000000000, 0.000000000000000000 ) ) ;
#11726=LINE ( 'NONE', #30748, #5859 ) ;
#11733=LINE ( 'NONE', #9858, #30240 ) ;
#11735=FACE_OUTER_BOUND ( 'NONE', #14334, .T. ) ;
#11746=ORIENTED_EDGE ( 'NONE', *, *, #17988, .T. ) ;
#11748=DIRECTION ( 'NONE',  ( 0.000000000000000000, 0.000000000000000000, 1.000000000000000000 ) ) ;
#11753=ORIENTED_EDGE ( 'NONE', *, *, #23330, .T. ) ;
#11754=CYLINDRICAL_SURFACE ( 'NONE', #9792, 0.7499999999999997780 ) ;
#11761=CARTESIAN_POINT ( 'NONE',  ( 9.033033306777456417, -0.9621688436939737077, 21.50000000000000000 ) ) ;
#11762=AXIS2_PLACEMENT_3D ( 'NONE', #604, #9981, #19786 ) ;
#11768=CARTESIAN_POINT ( 'NONE',  ( 0.000000000000000000, -2.435693370351110282E-15, 21.50000000000000355 ) ) ;
#11772=CARTESIAN_POINT ( 'NONE',  ( 8.268028093133368728, 3.763133143576462114, -1.500000000000001332 ) ) ;
#11778=DIRECTION ( 'NONE',  ( -0.000000000000000000, -0.000000000000000000, 1.000000000000000000 ) ) ;
#11793=ORIENTED_EDGE ( 'NONE', *, *, #28430, .T. ) ;
#11795=CARTESIAN_POINT ( 'NONE',  ( 3.683253992019827727, -8.303920738747228469, 13.22130136205108641 ) ) ;
#11798=CIRCLE ( 'NONE', #1832, 9.084132297865673777 ) ;
#11801=AXIS2_PLACEMENT_3D ( 'NONE', #8529, #15526, #24896 ) ;
#11802=FACE_OUTER_BOUND ( 'NONE', #9587, .T. ) ;
#11838=VERTEX_POINT ( 'NONE', #22187 ) ;
#11840=VERTEX_POINT ( 'NONE', #21714 ) ;
#11857=ORIENTED_EDGE ( 'NONE', *, *, #11460, .T. ) ;
#11858=AXIS2_PLACEMENT_3D ( 'NONE', #7398, #23753, #21723 ) ;
#11873=CIRCLE ( 'NONE', #28816, 12.18947652193948272 ) ;
#11876=DIRECTION ( 'NONE',  ( 0.000000000000000000, -1.132880637372608986E-16, 1.000000000000000000 ) ) ;
#11878=EDGE_CURVE ( 'NONE', #15766, #13097, #27499, .T. ) ;
#11879=ORIENTED_EDGE ( 'NONE', *, *, #1023, .T. ) ;
#11883=DIRECTION ( 'NONE',  ( 1.000000000000000000, 0.000000000000000000, -0.000000000000000000 ) ) ;
#11884=CIRCLE ( 'NONE', #13865, 0.7500000000000011102 ) ;
#11888=CARTESIAN_POINT ( 'NONE',  ( -0.6210184355500070197, 9.062880100047294718, 13.22130136205108997 ) ) ;
#11890=DIRECTION ( 'NONE',  ( 1.000000000000000000, 0.000000000000000000, 0.000000000000000000 ) ) ;
#11891=DIRECTION ( 'NONE',  ( 0.000000000000000000, -1.132880637372608986E-16, 1.000000000000000000 ) ) ;
#11893=( GEOMETRIC_REPRESENTATION_CONTEXT ( 3 ) GLOBAL_UNCERTAINTY_ASSIGNED_CONTEXT ( ( #27959 ) ) GLOBAL_UNIT_ASSIGNED_CONTEXT ( ( #4005, #5883, #23013 ) ) REPRESENTATION_CONTEXT ( 'NONE', 'WORKASPACE' ) );
#11898=CIRCLE ( 'NONE', #10903, 0.7499999999999997780 ) ;
#11900=AXIS2_PLACEMENT_3D ( 'NONE', #1447, #10326, #10960 ) ;
#11918=DIRECTION ( 'NONE',  ( -0.000000000000000000, 1.132880637372608986E-16, -1.000000000000000000 ) ) ;
#11949=ORIENTED_EDGE ( 'NONE', *, *, #1859, .F. ) ;
#11953=DIRECTION ( 'NONE',  ( 1.000000000000000000, 0.000000000000000000, 0.000000000000000000 ) ) ;
#11962=AXIS2_PLACEMENT_3D ( 'NONE', #25204, #8543, #30196 ) ;
#11966=DIRECTION ( 'NONE',  ( 0.000000000000000000, 1.132880637372608986E-16, -1.000000000000000000 ) ) ;
#11979=DIRECTION ( 'NONE',  ( -0.000000000000000000, 1.132880637372608986E-16, -1.000000000000000000 ) ) ;
#11985=CARTESIAN_POINT ( 'NONE',  ( 3.683253992019826839, -8.303920738747226693, -1.500000000000002665 ) ) ;
#11992=VECTOR ( 'NONE', #30848, 1000.000000000000000 ) ;
#12006=EDGE_LOOP ( 'NONE', ( #14464, #25704 ) ) ;
#12016=FACE_OUTER_BOUND ( 'NONE', #28851, .T. ) ;
#12027=CARTESIAN_POINT ( 'NONE',  ( 8.752572334588121450, -2.431858781452763019, -1.500000000000001998 ) ) ;
#12031=AXIS2_PLACEMENT_3D ( 'NONE', #30440, #11428, #21209 ) ;
#12059=EDGE_CURVE ( 'NONE', #1661, #16043, #19907, .T. ) ;
#12062=ORIENTED_EDGE ( 'NONE', *, *, #27609, .F. ) ;
#12063=ORIENTED_EDGE ( 'NONE', *, *, #13806, .T. ) ;
#12070=ORIENTED_EDGE ( 'NONE', *, *, #26562, .T. ) ;
#12072=VERTEX_POINT ( 'NONE', #13622 ) ;
#12075=ADVANCED_FACE ( 'NONE', ( #1744 ), #23704, .F. ) ;
#12087=CARTESIAN_POINT ( 'NONE',  ( 6.974883619896790954, 5.687793815610376669, 21.50000000000000000 ) ) ;
#12116=AXIS2_PLACEMENT_3D ( 'NONE', #9310, #18836, #28353 ) ;
#12117=VECTOR ( 'NONE', #22792, 1000.000000000000000 ) ;
#12129=DIRECTION ( 'NONE',  ( 1.000000000000000000, 0.000000000000000000, 0.000000000000000000 ) ) ;
#12164=ORIENTED_EDGE ( 'NONE', *, *, #9150, .F. ) ;
#12174=VERTEX_POINT ( 'NONE', #1420 ) ;
#12176=CARTESIAN_POINT ( 'NONE',  ( 0.000000000000000000, -2.435693370351110282E-15, 21.50000000000000355 ) ) ;
#12183=DIRECTION ( 'NONE',  ( -0.000000000000000000, -0.000000000000000000, 1.000000000000000000 ) ) ;
#12192=VERTEX_POINT ( 'NONE', #3752 ) ;
#12197=DIRECTION ( 'NONE',  ( -0.000000000000000000, 1.132880637372608986E-16, -1.000000000000000000 ) ) ;
#12198=CARTESIAN_POINT ( 'NONE',  ( 0.6237340761795171495, -8.999114229549588728, -1.500000000000002665 ) ) ;
#12201=DIRECTION ( 'NONE',  ( 0.000000000000000000, -1.132880637372608986E-16, 1.000000000000000000 ) ) ;
#12212=AXIS2_PLACEMENT_3D ( 'NONE', #10490, #15469, #15625 ) ;
#12222=DIRECTION ( 'NONE',  ( -0.000000000000000000, 1.132880637372608986E-16, -1.000000000000000000 ) ) ;
#12251=FACE_OUTER_BOUND ( 'NONE', #23966, .T. ) ;
#12258=LINE ( 'NONE', #17240, #17220 ) ;
#12268=AXIS2_PLACEMENT_3D ( 'NONE', #30401, #18413, #25873 ) ;
#12272=CARTESIAN_POINT ( 'NONE',  ( -4.390207617113899730, 7.856594496258241023, -3.621320343559650379 ) ) ;
#12275=AXIS2_PLACEMENT_3D ( 'NONE', #19743, #7283, #29272 ) ;
#12287=CYLINDRICAL_SURFACE ( 'NONE', #20602, 0.7500000000000006661 ) ;
#12292=CARTESIAN_POINT ( 'NONE',  ( -8.159193615868369776, 3.993622308618967498, -1.500000000000001332 ) ) ;
#12294=EDGE_LOOP ( 'NONE', ( #9559, #858, #2801, #21718 ) ) ;
#12299=ORIENTED_EDGE ( 'NONE', *, *, #18725, .F. ) ;
#12303=CIRCLE ( 'NONE', #9312, 9.084132297865673777 ) ;
#12310=CARTESIAN_POINT ( 'NONE',  ( 8.728722367416583694, -2.516121109503213216, -1.500000000000001998 ) ) ;
#12314=VERTEX_POINT ( 'NONE', #8732 ) ;
#12329=AXIS2_PLACEMENT_3D ( 'NONE', #29954, #18095, #27613 ) ;
#12334=ORIENTED_EDGE ( 'NONE', *, *, #12446, .F. ) ;
#12335=AXIS2_PLACEMENT_3D ( 'NONE', #608, #19631, #17936 ) ;
#12345=CARTESIAN_POINT ( 'NONE',  ( -2.959227181723746547, 8.499586724479465616, 21.50000000000000000 ) ) ;
#12353=CIRCLE ( 'NONE', #11858, 9.084132297865673777 ) ;
#12357=DIRECTION ( 'NONE',  ( 1.000000000000000000, 0.000000000000000000, 0.000000000000000000 ) ) ;
#12360=VERTEX_POINT ( 'NONE', #16058 ) ;
#12364=DIRECTION ( 'NONE',  ( 1.000000000000000000, 0.000000000000000000, 0.000000000000000000 ) ) ;
#12365=AXIS2_PLACEMENT_3D ( 'NONE', #6455, #10984, #11439 ) ;
#12372=CARTESIAN_POINT ( 'NONE',  ( 5.069257791428381843, -7.538175180318440027, 21.50000000000000000 ) ) ;
#12399=AXIS2_PLACEMENT_3D ( 'NONE', #17901, #27415, #6034 ) ;
#12404=CARTESIAN_POINT ( 'NONE',  ( -6.364020599487750118, 6.482337650448473099, 13.22130136205108819 ) ) ;
#12406=EDGE_CURVE ( 'NONE', #23519, #25108, #25407, .T. ) ;
#12416=DIRECTION ( 'NONE',  ( 1.000000000000000000, 0.000000000000000000, 0.000000000000000000 ) ) ;
#12420=ORIENTED_EDGE ( 'NONE', *, *, #16800, .F. ) ;
#12423=AXIS2_PLACEMENT_3D ( 'NONE', #4686, #14040, #6870 ) ;
#12440=VECTOR ( 'NONE', #23942, 1000.000000000000000 ) ;
#12446=EDGE_CURVE ( 'NONE', #6231, #19990, #28898, .T. ) ;
#12454=ADVANCED_FACE ( 'NONE', ( #22865 ), #20673, .F. ) ;
#12462=ORIENTED_EDGE ( 'NONE', *, *, #19927, .F. ) ;
#12467=CARTESIAN_POINT ( 'NONE',  ( -0.6210184355500071307, 9.062880100047296494, -1.500000000000000666 ) ) ;
#12476=DIRECTION ( 'NONE',  ( -0.000000000000000000, -0.000000000000000000, 1.000000000000000000 ) ) ;
#12479=DIRECTION ( 'NONE',  ( -0.000000000000000000, 1.132880637372608986E-16, -1.000000000000000000 ) ) ;
#12488=DIRECTION ( 'NONE',  ( 0.000000000000000000, 0.000000000000000000, 1.000000000000000000 ) ) ;
#12493=ORIENTED_EDGE ( 'NONE', *, *, #20040, .T. ) ;
#12498=PLANE ( 'NONE',  #14311 ) ;
#12511=CIRCLE ( 'NONE', #16483, 9.084132297865673777 ) ;
#12530=DIRECTION ( 'NONE',  ( -9.830099697201897928E-15, 1.000000000000000000, 0.000000000000000000 ) ) ;
#12535=ORIENTED_EDGE ( 'NONE', *, *, #18370, .F. ) ;
#12539=ORIENTED_EDGE ( 'NONE', *, *, #5452, .T. ) ;
#12545=CARTESIAN_POINT ( 'NONE',  ( -6.812559277181930106, 5.881244434206302607, -3.621320343559650379 ) ) ;
#12550=CARTESIAN_POINT ( 'NONE',  ( -6.224883619896829146, -5.687793815610328707, -1.500000000000002220 ) ) ;
#12554=AXIS2_PLACEMENT_3D ( 'NONE', #30655, #6972, #24719 ) ;
#12559=DIRECTION ( 'NONE',  ( -0.000000000000000000, -0.000000000000000000, 1.000000000000000000 ) ) ;
#12570=CARTESIAN_POINT ( 'NONE',  ( 5.881244434206234217, 6.812559277181991391, -3.621320343559650379 ) ) ;
#12580=EDGE_CURVE ( 'NONE', #9872, #23362, #13467, .T. ) ;
#12589=LINE ( 'NONE', #8209, #8310 ) ;
#12593=DIRECTION ( 'NONE',  ( 0.000000000000000000, -1.132880637372608986E-16, 1.000000000000000000 ) ) ;
#12594=ORIENTED_EDGE ( 'NONE', *, *, #11311, .T. ) ;
#12612=DIRECTION ( 'NONE',  ( 2.312964634635743450E-15, 1.000000000000000000, 0.000000000000000000 ) ) ;
#12617=EDGE_LOOP ( 'NONE', ( #24318, #13132, #23982 ) ) ;
#12623=ADVANCED_FACE ( 'NONE', ( #30493 ), #2257, .F. ) ;
#12629=CYLINDRICAL_SURFACE ( 'NONE', #5886, 9.084132297865673777 ) ;
#12636=VERTEX_POINT ( 'NONE', #8834 ) ;
#12638=LINE ( 'NONE', #469, #1183 ) ;
#12673=EDGE_LOOP ( 'NONE', ( #21341, #28278 ) ) ;
#12696=LINE ( 'NONE', #2666, #7906 ) ;
#12701=CARTESIAN_POINT ( 'NONE',  ( -8.817355867515827228, -2.185336383880175593, 13.22130136205108819 ) ) ;
#12713=ORIENTED_EDGE ( 'NONE', *, *, #4434, .T. ) ;
#12757=CARTESIAN_POINT ( 'NONE',  ( -3.858906612435654804, -7.730328572437724866, -1.500000000000002665 ) ) ;
#12758=AXIS2_PLACEMENT_3D ( 'NONE', #29967, #20447, #30112 ) ;
#12766=( NAMED_UNIT ( * ) PLANE_ANGLE_UNIT ( ) SI_UNIT ( $, .RADIAN. ) );
#12786=CARTESIAN_POINT ( 'NONE',  ( -1.687027447297492211, -8.840471615930066918, -1.500000000000002665 ) ) ;
#12787=DIRECTION ( 'NONE',  ( 0.000000000000000000, -1.132880637372608986E-16, 1.000000000000000000 ) ) ;
#12798=EDGE_CURVE ( 'NONE', #4256, #12192, #4494, .T. ) ;
#12802=CIRCLE ( 'NONE', #30224, 9.084132297865673777 ) ;
#12812=LINE ( 'NONE', #488, #26534 ) ;
#12832=CARTESIAN_POINT ( 'NONE',  ( 0.000000000000000000, 1.699320956058915452E-16, -1.500000000000001776 ) ) ;
#12837=CIRCLE ( 'NONE', #30252, 0.7500000000000002220 ) ;
#12850=PLANE ( 'NONE',  #28318 ) ;
#12851=CIRCLE ( 'NONE', #23291, 0.7500000000000011102 ) ;
#12857=CARTESIAN_POINT ( 'NONE',  ( -4.390207617113899730, 7.856594496258241023, 21.50000000000000000 ) ) ;
#12858=DIRECTION ( 'NONE',  ( 0.000000000000000000, 1.132880637372608986E-16, -1.000000000000000000 ) ) ;
#12865=EDGE_CURVE ( 'NONE', #30279, #24466, #3810, .T. ) ;
#12893=EDGE_CURVE ( 'NONE', #7139, #20169, #29417, .T. ) ;
#12897=CIRCLE ( 'NONE', #30310, 0.7500000000000006661 ) ;
#12907=ORIENTED_EDGE ( 'NONE', *, *, #22685, .T. ) ;
#12913=VECTOR ( 'NONE', #22706, 1000.000000000000000 ) ;
#12917=CARTESIAN_POINT ( 'NONE',  ( 0.000000000000000000, -2.435693370351110282E-15, 21.50000000000000355 ) ) ;
#12930=DIRECTION ( 'NONE',  ( 0.000000000000000000, 1.000000000000000000, 0.000000000000000000 ) ) ;
#12946=ORIENTED_EDGE ( 'NONE', *, *, #12406, .T. ) ;
#12948=DIRECTION ( 'NONE',  ( 0.000000000000000000, 0.000000000000000000, 1.000000000000000000 ) ) ;
#12958=EDGE_LOOP ( 'NONE', ( #6884, #16055 ) ) ;
#12974=DIRECTION ( 'NONE',  ( -0.000000000000000000, 1.132880637372608986E-16, -1.000000000000000000 ) ) ;
#12975=CIRCLE ( 'NONE', #11483, 0.7500000000000007772 ) ;
#12990=ORIENTED_EDGE ( 'NONE', *, *, #24261, .T. ) ;
#12998=VECTOR ( 'NONE', #13689, 1000.000000000000000 ) ;
#13005=DIRECTION ( 'NONE',  ( 2.312964634635740689E-15, 1.000000000000000000, 0.000000000000000000 ) ) ;
#13019=AXIS2_PLACEMENT_3D ( 'NONE', #26103, #28606, #16740 ) ;
#13021=AXIS2_PLACEMENT_3D ( 'NONE', #17292, #19480, #919 ) ;
#13028=CARTESIAN_POINT ( 'NONE',  ( 2.959227181723801170, -8.499586724479446076, 21.50000000000000000 ) ) ;
#13029=ORIENTED_EDGE ( 'NONE', *, *, #9962, .T. ) ;
#13031=CARTESIAN_POINT ( 'NONE',  ( -8.795879380940577974, -2.270234684139648351, 21.50000000000000000 ) ) ;
#13054=PLANE ( 'NONE',  #26293 ) ;
#13055=DIRECTION ( 'NONE',  ( 1.000000000000000000, 0.000000000000000000, 0.000000000000000000 ) ) ;
#13066=EDGE_CURVE ( 'NONE', #26044, #19148, #15965, .T. ) ;
#13081=ORIENTED_EDGE ( 'NONE', *, *, #10365, .T. ) ;
#13083=DIRECTION ( 'NONE',  ( 0.000000000000000000, 0.000000000000000000, 1.000000000000000000 ) ) ;
#13097=VERTEX_POINT ( 'NONE', #23282 ) ;
#13109=EDGE_LOOP ( 'NONE', ( #29509, #299, #18217, #3207 ) ) ;
#13110=CARTESIAN_POINT ( 'NONE',  ( 1.836970198721034716E-15, -15.00000000000005862, 117.5000000000000000 ) ) ;
#13126=FACE_OUTER_BOUND ( 'NONE', #27982, .T. ) ;
#13132=ORIENTED_EDGE ( 'NONE', *, *, #22557, .F. ) ;
#13152=ORIENTED_EDGE ( 'NONE', *, *, #11664, .T. ) ;
#13153=DIRECTION ( 'NONE',  ( 0.000000000000000000, 0.000000000000000000, 1.000000000000000000 ) ) ;
#13161=ORIENTED_EDGE ( 'NONE', *, *, #2096, .T. ) ;
#13169=DIRECTION ( 'NONE',  ( -0.000000000000000000, -0.000000000000000000, 1.000000000000000000 ) ) ;
#13177=FACE_OUTER_BOUND ( 'NONE', #25872, .T. ) ;
#13178=EDGE_LOOP ( 'NONE', ( #10786, #16686, #18097, #20701 ) ) ;
#13200=FACE_OUTER_BOUND ( 'NONE', #15711, .T. ) ;
#13202=CYLINDRICAL_SURFACE ( 'NONE', #4565, 0.7500000000000003331 ) ;
#13203=DIRECTION ( 'NONE',  ( -0.000000000000000000, -0.000000000000000000, 1.000000000000000000 ) ) ;
#13204=EDGE_CURVE ( 'NONE', #8467, #20812, #11427, .T. ) ;
#13209=CYLINDRICAL_SURFACE ( 'NONE', #23514, 12.18947652193948272 ) ;
#13211=EDGE_CURVE ( 'NONE', #17470, #14477, #30822, .T. ) ;
#13215=CARTESIAN_POINT ( 'NONE',  ( -8.413215745754975217, 3.196529495465474380, 21.50000000000000000 ) ) ;
#13219=PLANE ( 'NONE',  #22844 ) ;
#13220=CYLINDRICAL_SURFACE ( 'NONE', #19657, 0.7500000000000006661 ) ;
#13221=EDGE_CURVE ( 'NONE', #28571, #28301, #44, .T. ) ;
#13233=ORIENTED_EDGE ( 'NONE', *, *, #6711, .T. ) ;
#13234=DIRECTION ( 'NONE',  ( 1.000000000000000000, 0.000000000000000000, 0.000000000000000000 ) ) ;
#13236=ORIENTED_EDGE ( 'NONE', *, *, #11664, .F. ) ;
#13247=DIRECTION ( 'NONE',  ( -0.000000000000000000, -0.000000000000000000, 1.000000000000000000 ) ) ;
#13252=ORIENTED_EDGE ( 'NONE', *, *, #21561, .T. ) ;
#13256=FACE_OUTER_BOUND ( 'NONE', #21321, .T. ) ;
#13260=CIRCLE ( 'NONE', #12268, 9.084132297865673777 ) ;
#13262=DIRECTION ( 'NONE',  ( 0.000000000000000000, 1.000000000000000000, 1.193512090021232842E-16 ) ) ;
#13270=ORIENTED_EDGE ( 'NONE', *, *, #2096, .F. ) ;
#13280=VECTOR ( 'NONE', #57, 1000.000000000000000 ) ;
#13296=LINE ( 'NONE', #6424, #12117 ) ;
#13299=CARTESIAN_POINT ( 'NONE',  ( -9.056472324687613096, -0.7083562926194844067, 13.22130136205108819 ) ) ;
#13303=DIRECTION ( 'NONE',  ( 0.000000000000000000, -1.132880637372608986E-16, 1.000000000000000000 ) ) ;
#13306=ORIENTED_EDGE ( 'NONE', *, *, #2750, .T. ) ;
#13315=DIRECTION ( 'NONE',  ( 0.000000000000000000, 0.000000000000000000, 1.000000000000000000 ) ) ;
#13316=VECTOR ( 'NONE', #6435, 1000.000000000000000 ) ;
#13317=CARTESIAN_POINT ( 'NONE',  ( 7.730328572437743517, -4.608906612435629491, -3.621320343559650379 ) ) ;
#13325=DIRECTION ( 'NONE',  ( 1.000000000000000000, 0.000000000000000000, 0.000000000000000000 ) ) ;
#13342=AXIS2_PLACEMENT_3D ( 'NONE', #10256, #29300, #7941 ) ;
#13347=EDGE_CURVE ( 'NONE', #2272, #29438, #21340, .T. ) ;
#13360=CIRCLE ( 'NONE', #22806, 9.084132297865673777 ) ;
#13362=AXIS2_PLACEMENT_3D ( 'NONE', #9578, #26257, #2239 ) ;
#13364=CYLINDRICAL_SURFACE ( 'NONE', #26964, 0.7500000000000002220 ) ;
#13365=CARTESIAN_POINT ( 'NONE',  ( 2.959227181723801170, -8.499586724479446076, -1.500000000000002665 ) ) ;
#13368=FACE_OUTER_BOUND ( 'NONE', #30841, .T. ) ;
#13370=VERTEX_POINT ( 'NONE', #25134 ) ;
#13376=EDGE_LOOP ( 'NONE', ( #14469, #5424, #29606, #12713 ) ) ;
#13378=AXIS2_PLACEMENT_3D ( 'NONE', #19133, #23800, #9930 ) ;
#13381=DIRECTION ( 'NONE',  ( 0.000000000000000000, 0.000000000000000000, 1.000000000000000000 ) ) ;
#13383=ORIENTED_EDGE ( 'NONE', *, *, #27045, .T. ) ;
#13385=CARTESIAN_POINT ( 'NONE',  ( 0.000000000000000000, 1.699320956058915452E-16, -1.500000000000001776 ) ) ;
#13387=CARTESIAN_POINT ( 'NONE',  ( -6.224883619896829146, -5.687793815610328707, -3.621320343559650379 ) ) ;
#13389=LINE ( 'NONE', #22880, #384 ) ;
#13392=ADVANCED_FACE ( 'NONE', ( #804 ), #3305, .F. ) ;
#13398=EDGE_CURVE ( 'NONE', #191, #4424, #1939, .T. ) ;
#13408=DIRECTION ( 'NONE',  ( 0.000000000000000000, 1.000000000000000000, 0.000000000000000000 ) ) ;
#13412=EDGE_CURVE ( 'NONE', #27939, #7334, #22478, .T. ) ;
#13414=CIRCLE ( 'NONE', #15386, 9.084132297865673777 ) ;
#13417=ORIENTED_EDGE ( 'NONE', *, *, #1927, .F. ) ;
#13422=ORIENTED_EDGE ( 'NONE', *, *, #19089, .F. ) ;
#13426=CARTESIAN_POINT ( 'NONE',  ( -6.980328572437709767, 4.608906612435681005, -3.621320343559650379 ) ) ;
#13428=FACE_OUTER_BOUND ( 'NONE', #1941, .T. ) ;
#13431=ORIENTED_EDGE ( 'NONE', *, *, #868, .F. ) ;
#13436=ADVANCED_FACE ( 'NONE', ( #30276 ), #11560, .F. ) ;
#13462=DIRECTION ( 'NONE',  ( 1.000000000000000000, 0.000000000000000000, 0.000000000000000000 ) ) ;
#13464=EDGE_CURVE ( 'NONE', #25155, #28714, #16879, .T. ) ;
#13465=ORIENTED_EDGE ( 'NONE', *, *, #1825, .T. ) ;
#13467=CIRCLE ( 'NONE', #8504, 9.084132297865673777 ) ;
#13477=DIRECTION ( 'NONE',  ( 1.000000000000000000, 0.000000000000000000, 0.000000000000000000 ) ) ;
#13480=AXIS2_PLACEMENT_3D ( 'NONE', #21375, #14359, #12 ) ;
#13498=DIRECTION ( 'NONE',  ( 0.000000000000000000, 1.000000000000000000, 1.193512090021232842E-16 ) ) ;
#13514=DIRECTION ( 'NONE',  ( 0.000000000000000000, 1.000000000000000000, 0.000000000000000000 ) ) ;
#13515=AXIS2_PLACEMENT_3D ( 'NONE', #18910, #23559, #26388 ) ;
#13518=CARTESIAN_POINT ( 'NONE',  ( -0.6237340761795794331, 8.999114229549594057, -1.500000000000000888 ) ) ;
#13522=DIRECTION ( 'NONE',  ( 0.000000000000000000, 1.000000000000000000, 0.000000000000000000 ) ) ;
#13523=LINE ( 'NONE', #26831, #4432 ) ;
#13529=DIRECTION ( 'NONE',  ( 0.000000000000000000, -1.132880637372608986E-16, 1.000000000000000000 ) ) ;
#13531=SHAPE_REPRESENTATION_RELATIONSHIP ( 'NONE' , 'NONE' ,  #23229, #5063 ) ;
#13535=ORIENTED_EDGE ( 'NONE', *, *, #24634, .T. ) ;
#13539=AXIS2_PLACEMENT_3D ( 'NONE', #22956, #22808, #1746 ) ;
#13559=AXIS2_PLACEMENT_3D ( 'NONE', #28345, #21616, #28798 ) ;
#13566=CARTESIAN_POINT ( 'NONE',  ( 0.000000000000000000, 12.18947652193948272, -87.50000000000000000 ) ) ;
#13568=LINE ( 'NONE', #28050, #4704 ) ;
#13581=AXIS2_PLACEMENT_3D ( 'NONE', #14865, #15165, #24380 ) ;
#13600=ORIENTED_EDGE ( 'NONE', *, *, #6309, .F. ) ;
#13606=LINE ( 'NONE', #30121, #29709 ) ;
#13613=EDGE_CURVE ( 'NONE', #29162, #549, #8691, .T. ) ;
#13617=ORIENTED_EDGE ( 'NONE', *, *, #5907, .F. ) ;
#13620=ORIENTED_EDGE ( 'NONE', *, *, #20899, .T. ) ;
#13622=CARTESIAN_POINT ( 'NONE',  ( -8.197313248159920462, 3.914781618004780306, 21.50000000000000000 ) ) ;
#13635=EDGE_CURVE ( 'NONE', #1968, #24589, #15858, .T. ) ;
#13652=CARTESIAN_POINT ( 'NONE',  ( 6.482337650448408262, 6.364020599487814955, 21.50000000000000000 ) ) ;
#13673=CARTESIAN_POINT ( 'NONE',  ( 8.999114229549594057, -0.1262659238204522361, -1.500000000000001776 ) ) ;
#13681=DIRECTION ( 'NONE',  ( 0.000000000000000000, 1.000000000000000000, 0.000000000000000000 ) ) ;
#13689=DIRECTION ( 'NONE',  ( -0.000000000000000000, -0.000000000000000000, 1.000000000000000000 ) ) ;
#13690=ORIENTED_EDGE ( 'NONE', *, *, #29510, .T. ) ;
#13691=CARTESIAN_POINT ( 'NONE',  ( -0.1262659238204836554, -8.999114229549588728, -1.500000000000002665 ) ) ;
#13693=CARTESIAN_POINT ( 'NONE',  ( -3.683253992019774881, 8.303920738747249786, -1.500000000000000888 ) ) ;
#13697=CARTESIAN_POINT ( 'NONE',  ( -7.538175180318458679, -5.069257791428355198, 21.50000000000000000 ) ) ;
#13698=DIRECTION ( 'NONE',  ( 0.000000000000000000, 1.000000000000000000, 0.000000000000000000 ) ) ;
#13704=CARTESIAN_POINT ( 'NONE',  ( 5.141690706682880752, -7.488956955540417404, 21.50000000000000000 ) ) ;
#13722=ORIENTED_EDGE ( 'NONE', *, *, #29867, .T. ) ;
#13729=CYLINDRICAL_SURFACE ( 'NONE', #8362, 0.7500000000000004441 ) ;
#13731=EDGE_LOOP ( 'NONE', ( #14488, #8183, #11425, #30734 ) ) ;
#13734=DIRECTION ( 'NONE',  ( 1.156482317317870344E-15, 1.000000000000000000, 0.000000000000000000 ) ) ;
#13744=ADVANCED_FACE ( 'NONE', ( #15694 ), #13219, .F. ) ;
#13771=DIRECTION ( 'NONE',  ( 0.000000000000000000, -1.132880637372608986E-16, 1.000000000000000000 ) ) ;
#13778=ADVANCED_FACE ( 'NONE', ( #12251 ), #17398, .F. ) ;
#13779=AXIS2_PLACEMENT_3D ( 'NONE', #11198, #1990, #23494 ) ;
#13799=EDGE_CURVE ( 'NONE', #29438, #3254, #4460, .T. ) ;
#13804=DIRECTION ( 'NONE',  ( -0.000000000000000000, 1.132880637372608986E-16, -1.000000000000000000 ) ) ;
#13805=ORIENTED_EDGE ( 'NONE', *, *, #23301, .F. ) ;
#13806=EDGE_CURVE ( 'NONE', #23362, #28205, #19425, .T. ) ;
#13817=DIRECTION ( 'NONE',  ( 0.000000000000000000, -1.132880637372608986E-16, 1.000000000000000000 ) ) ;
#13855=DIRECTION ( 'NONE',  ( 0.000000000000000000, 0.000000000000000000, 1.000000000000000000 ) ) ;
#13865=AXIS2_PLACEMENT_3D ( 'NONE', #27540, #1943, #18335 ) ;
#13872=DIRECTION ( 'NONE',  ( 0.000000000000000000, 0.000000000000000000, 1.000000000000000000 ) ) ;
#13873=ORIENTED_EDGE ( 'NONE', *, *, #27310, .F. ) ;
#13875=AXIS2_PLACEMENT_3D ( 'NONE', #29226, #12858, #26897 ) ;
#13878=EDGE_LOOP ( 'NONE', ( #27455, #24200, #26484, #22069 ) ) ;
#13917=CARTESIAN_POINT ( 'NONE',  ( 0.000000000000000000, -2.435693370351110282E-15, 21.50000000000000355 ) ) ;
#13919=LINE ( 'NONE', #24026, #30255 ) ;
#13934=EDGE_CURVE ( 'NONE', #11358, #15951, #17741, .T. ) ;
#13967=CIRCLE ( 'NONE', #28932, 0.7500000000000006661 ) ;
#13974=LINE ( 'NONE', #18656, #25844 ) ;
#13979=EDGE_CURVE ( 'NONE', #2547, #28904, #26571, .T. ) ;
#13989=EDGE_CURVE ( 'NONE', #21542, #11840, #1163, .T. ) ;
#13991=AXIS2_PLACEMENT_3D ( 'NONE', #27611, #28204, #6836 ) ;
#13993=ORIENTED_EDGE ( 'NONE', *, *, #13204, .F. ) ;
#14000=DIRECTION ( 'NONE',  ( 0.000000000000000000, 1.000000000000000000, 0.000000000000000000 ) ) ;
#14002=ADVANCED_FACE ( 'NONE', ( #4574 ), #4423, .F. ) ;
#14003=EDGE_CURVE ( 'NONE', #12360, #7713, #9560, .T. ) ;
#14005=PLANE ( 'NONE',  #5618 ) ;
#14008=DIRECTION ( 'NONE',  ( -0.000000000000000000, 1.132880637372608986E-16, -1.000000000000000000 ) ) ;
#14012=DIRECTION ( 'NONE',  ( 1.000000000000000000, 0.000000000000000000, 0.000000000000000000 ) ) ;
#14017=ORIENTED_EDGE ( 'NONE', *, *, #22387, .T. ) ;
#14024=AXIS2_PLACEMENT_3D ( 'NONE', #18349, #25822, #28152 ) ;
#14036=DIRECTION ( 'NONE',  ( 1.000000000000000000, 0.000000000000000000, 0.000000000000000000 ) ) ;
#14040=DIRECTION ( 'NONE',  ( 0.000000000000000000, 0.000000000000000000, 1.000000000000000000 ) ) ;
#14055=FACE_OUTER_BOUND ( 'NONE', #29757, .T. ) ;
#14057=DIRECTION ( 'NONE',  ( 1.000000000000000000, 0.000000000000000000, -0.000000000000000000 ) ) ;
#14059=ORIENTED_EDGE ( 'NONE', *, *, #11135, .F. ) ;
#14063=DIRECTION ( 'NONE',  ( 1.000000000000000000, 0.000000000000000000, 0.000000000000000000 ) ) ;
#14075=AXIS2_PLACEMENT_3D ( 'NONE', #3341, #24699, #10367 ) ;
#14098=CARTESIAN_POINT ( 'NONE',  ( -2.431858781452794549, -8.752572334588112568, -1.500000000000002887 ) ) ;
#14110=CARTESIAN_POINT ( 'NONE',  ( 1.687027447297431371, 8.840471615930075799, 21.50000000000000000 ) ) ;
#14119=ORIENTED_EDGE ( 'NONE', *, *, #19172, .T. ) ;
#14120=AXIS2_PLACEMENT_3D ( 'NONE', #14505, #22134, #9672 ) ;
#14124=VERTEX_POINT ( 'NONE', #193 ) ;
#14126=DIRECTION ( 'NONE',  ( 0.000000000000000000, 1.000000000000000000, 1.193512090021232842E-16 ) ) ;
#14142=DIRECTION ( 'NONE',  ( 1.000000000000000000, 0.000000000000000000, 0.000000000000000000 ) ) ;
#14147=ORIENTED_EDGE ( 'NONE', *, *, #11034, .T. ) ;
#14152=ORIENTED_EDGE ( 'NONE', *, *, #2678, .F. ) ;
#14160=CARTESIAN_POINT ( 'NONE',  ( 1.492780340587499928E-15, -12.18947652193948272, -87.50000000000000000 ) ) ;
#14175=DIRECTION ( 'NONE',  ( 0.000000000000000000, -1.132880637372608986E-16, 1.000000000000000000 ) ) ;
#14191=CARTESIAN_POINT ( 'NONE',  ( -5.687793815610304726, 6.974883619896852238, 21.50000000000000000 ) ) ;
#14196=ADVANCED_FACE ( 'NONE', ( #28592 ), #24367, .F. ) ;
#14212=ORIENTED_EDGE ( 'NONE', *, *, #25949, .F. ) ;
#14213=DIRECTION ( 'NONE',  ( 0.000000000000000000, 0.000000000000000000, 1.000000000000000000 ) ) ;
#14218=VERTEX_POINT ( 'NONE', #12372 ) ;
#14233=ORIENTED_EDGE ( 'NONE', *, *, #21494, .T. ) ;
#14249=CYLINDRICAL_SURFACE ( 'NONE', #10425, 0.7500000000000006661 ) ;
#14256=CIRCLE ( 'NONE', #29216, 9.084132297865673777 ) ;
#14265=EDGE_CURVE ( 'NONE', #8229, #1903, #14313, .T. ) ;
#14275=ADVANCED_FACE ( 'NONE', ( #22023 ), #3781, .T. ) ;
#14278=CIRCLE ( 'NONE', #4315, 0.7500000000000006661 ) ;
#14290=CARTESIAN_POINT ( 'NONE',  ( -8.413215745754975217, 3.196529495465474380, -1.500000000000001332 ) ) ;
#14293=CARTESIAN_POINT ( 'NONE',  ( 5.687793815610356241, -6.974883619896809606, -1.500000000000002665 ) ) ;
#14311=AXIS2_PLACEMENT_3D ( 'NONE', #7656, #5152, #14973 ) ;
#14312=DIRECTION ( 'NONE',  ( 1.000000000000000000, 0.000000000000000000, 0.000000000000000000 ) ) ;
#14313=CIRCLE ( 'NONE', #6286, 0.7500000000000006661 ) ;
#14318=EDGE_CURVE ( 'NONE', #11562, #34, #11511, .T. ) ;
#14321=EDGE_CURVE ( 'NONE', #17470, #9984, #22636, .T. ) ;
#14326=AXIS2_PLACEMENT_3D ( 'NONE', #25926, #20485, #3965 ) ;
#14334=EDGE_LOOP ( 'NONE', ( #10822, #10049, #14233, #24335 ) ) ;
#14345=DIRECTION ( 'NONE',  ( 1.000000000000000000, 0.000000000000000000, -0.000000000000000000 ) ) ;
#14359=DIRECTION ( 'NONE',  ( 0.000000000000000000, 0.000000000000000000, 1.000000000000000000 ) ) ;
#14373=DIRECTION ( 'NONE',  ( 0.000000000000000000, 1.000000000000000000, 0.000000000000000000 ) ) ;
#14380=AXIS2_PLACEMENT_3D ( 'NONE', #13365, #15206, #8681 ) ;
#14385=DIRECTION ( 'NONE',  ( 0.000000000000000000, -1.132880637372608986E-16, 1.000000000000000000 ) ) ;
#14386=CARTESIAN_POINT ( 'NONE',  ( 0.000000000000000000, -2.435693370351110282E-15, 21.50000000000000355 ) ) ;
#14391=AXIS2_PLACEMENT_3D ( 'NONE', #13215, #18047, #27562 ) ;
#14409=AXIS2_PLACEMENT_3D ( 'NONE', #1509, #17715, #8536 ) ;
#14411=ORIENTED_EDGE ( 'NONE', *, *, #6087, .F. ) ;
#14431=ORIENTED_EDGE ( 'NONE', *, *, #28215, .F. ) ;
#14432=EDGE_LOOP ( 'NONE', ( #28614, #30639 ) ) ;
#14464=ORIENTED_EDGE ( 'NONE', *, *, #18423, .F. ) ;
#14467=DIRECTION ( 'NONE',  ( 0.000000000000000000, 1.000000000000000000, 1.193512090021232842E-16 ) ) ;
#14469=ORIENTED_EDGE ( 'NONE', *, *, #22137, .F. ) ;
#14472=ORIENTED_EDGE ( 'NONE', *, *, #29614, .F. ) ;
#14477=VERTEX_POINT ( 'NONE', #27794 ) ;
#14486=CARTESIAN_POINT ( 'NONE',  ( -6.980328572437709767, 4.608906612435681005, 21.50000000000000000 ) ) ;
#14488=ORIENTED_EDGE ( 'NONE', *, *, #19693, .F. ) ;
#14490=AXIS2_PLACEMENT_3D ( 'NONE', #26728, #27042, #13005 ) ;
#14494=CYLINDRICAL_SURFACE ( 'NONE', #14822, 0.7500000000000002220 ) ;
#14497=ORIENTED_EDGE ( 'NONE', *, *, #19128, .F. ) ;
#14505=CARTESIAN_POINT ( 'NONE',  ( -2.959227181723746547, 8.499586724479465616, -1.500000000000000888 ) ) ;
#14541=ADVANCED_FACE ( 'NONE', ( #21047 ), #25896, .F. ) ;
#14550=DIRECTION ( 'NONE',  ( 0.000000000000000000, 1.132880637372608986E-16, -1.000000000000000000 ) ) ;
#14557=ORIENTED_EDGE ( 'NONE', *, *, #14318, .T. ) ;
#14573=ORIENTED_EDGE ( 'NONE', *, *, #4389, .F. ) ;
#14578=CIRCLE ( 'NONE', #4663, 0.7499999999999997780 ) ;
#14579=AXIS2_PLACEMENT_3D ( 'NONE', #17801, #27315, #30104 ) ;
#14590=ORIENTED_EDGE ( 'NONE', *, *, #4057, .F. ) ;
#14596=CARTESIAN_POINT ( 'NONE',  ( 8.884323311075775109, 1.438332125858202692, -3.621320343559650379 ) ) ;
#14605=ORIENTED_EDGE ( 'NONE', *, *, #7875, .F. ) ;
#14627=DIRECTION ( 'NONE',  ( 0.000000000000000000, -1.132880637372608986E-16, 1.000000000000000000 ) ) ;
#14632=DIRECTION ( 'NONE',  ( 0.000000000000000000, -1.132880637372608986E-16, 1.000000000000000000 ) ) ;
#14661=EDGE_CURVE ( 'NONE', #20812, #28337, #12638, .T. ) ;
#14662=EDGE_LOOP ( 'NONE', ( #1492, #30095, #23743 ) ) ;
#14668=DIRECTION ( 'NONE',  ( 1.000000000000000000, 0.000000000000000000, 0.000000000000000000 ) ) ;
#14676=LINE ( 'NONE', #15138, #15860 ) ;
#14683=EDGE_CURVE ( 'NONE', #9984, #19691, #22091, .T. ) ;
#14698=AXIS2_PLACEMENT_3D ( 'NONE', #12176, #26206, #24330 ) ;
#14701=EDGE_CURVE ( 'NONE', #15766, #6758, #8668, .T. ) ;
#14711=VERTEX_POINT ( 'NONE', #1694 ) ;
#14718=VERTEX_POINT ( 'NONE', #20261 ) ;
#14727=ORIENTED_EDGE ( 'NONE', *, *, #23113, .F. ) ;
#14759=VERTEX_POINT ( 'NONE', #15419 ) ;
#14784=AXIS2_PLACEMENT_3D ( 'NONE', #18296, #7042, #11890 ) ;
#14785=ORIENTED_EDGE ( 'NONE', *, *, #11460, .F. ) ;
#14786=CIRCLE ( 'NONE', #10817, 0.7499999999999997780 ) ;
#14792=CARTESIAN_POINT ( 'NONE',  ( -3.914781618004754105, -8.197313248159934673, 21.50000000000000000 ) ) ;
#14799=AXIS2_PLACEMENT_3D ( 'NONE', #7204, #28575, #7370 ) ;
#14813=ORIENTED_EDGE ( 'NONE', *, *, #4473, .F. ) ;
#14814=CARTESIAN_POINT ( 'NONE',  ( -8.999114229549592281, 0.1262659238205133538, -1.500000000000001776 ) ) ;
#14822=AXIS2_PLACEMENT_3D ( 'NONE', #23994, #28855, #18878 ) ;
#14823=DIRECTION ( 'NONE',  ( 0.000000000000000000, 0.000000000000000000, 1.000000000000000000 ) ) ;
#14837=LINE ( 'NONE', #24349, #18252 ) ;
#14839=CARTESIAN_POINT ( 'NONE',  ( -0.6237340761795794331, 8.999114229549594057, 21.50000000000000000 ) ) ;
#14844=CARTESIAN_POINT ( 'NONE',  ( -4.937793815610304726, 6.974883619896852238, -3.621320343559650379 ) ) ;
#14865=CARTESIAN_POINT ( 'NONE',  ( 0.000000000000000000, -2.435693370351110282E-15, 21.50000000000000355 ) ) ;
#14871=EDGE_LOOP ( 'NONE', ( #12462, #17301, #15721, #13600 ) ) ;
#14883=ADVANCED_FACE ( 'NONE', ( #13256 ), #1404, .F. ) ;
#14897=FACE_OUTER_BOUND ( 'NONE', #12294, .T. ) ;
#14898=EDGE_CURVE ( 'NONE', #4424, #25108, #16190, .T. ) ;
#14902=VECTOR ( 'NONE', #22446, 1000.000000000000000 ) ;
#14904=FACE_OUTER_BOUND ( 'NONE', #1454, .T. ) ;
#14913=ORIENTED_EDGE ( 'NONE', *, *, #28215, .T. ) ;
#14955=ORIENTED_EDGE ( 'NONE', *, *, #15129, .T. ) ;
#14959=EDGE_LOOP ( 'NONE', ( #20320, #10606 ) ) ;
#14965=AXIS2_PLACEMENT_3D ( 'NONE', #3906, #23372, #6542 ) ;
#14972=VERTEX_POINT ( 'NONE', #22410 ) ;
#14973=DIRECTION ( 'NONE',  ( 1.000000000000000000, 0.000000000000000000, -0.000000000000000000 ) ) ;
#14977=CARTESIAN_POINT ( 'NONE',  ( 0.1262659238204208167, 8.999114229549594057, -3.621320343559650379 ) ) ;
#14997=LINE ( 'NONE', #17820, #15259 ) ;
#15006=CARTESIAN_POINT ( 'NONE',  ( 0.000000000000000000, 10.00000000000000888, 157.4999999999999716 ) ) ;
#15016=CARTESIAN_POINT ( 'NONE',  ( -8.499586724479453181, -2.959227181723774525, -1.500000000000002220 ) ) ;
#15017=LINE ( 'NONE', #12701, #3309 ) ;
#15024=AXIS2_PLACEMENT_3D ( 'NONE', #19510, #17484, #14668 ) ;
#15031=ORIENTED_EDGE ( 'NONE', *, *, #24313, .F. ) ;
#15036=CARTESIAN_POINT ( 'NONE',  ( -7.341751895053199917, 5.349779314757666882, -1.500000000000001110 ) ) ;
#15043=ORIENTED_EDGE ( 'NONE', *, *, #6512, .T. ) ;
#15055=AXIS2_PLACEMENT_3D ( 'NONE', #27528, #6302, #18018 ) ;
#15061=FACE_OUTER_BOUND ( 'NONE', #9710, .T. ) ;
#15073=EDGE_LOOP ( 'NONE', ( #2663, #9832, #25732, #1522, #1271 ) ) ;
#15076=ORIENTED_EDGE ( 'NONE', *, *, #26840, .T. ) ;
#15079=DIRECTION ( 'NONE',  ( -0.000000000000000000, 1.132880637372608986E-16, -1.000000000000000000 ) ) ;
#15094=DIRECTION ( 'NONE',  ( 1.000000000000000000, 0.000000000000000000, 0.000000000000000000 ) ) ;
#15102=ADVANCED_FACE ( 'NONE', ( #24123 ), #12287, .F. ) ;
#15110=DIRECTION ( 'NONE',  ( 0.000000000000000000, -1.132880637372608986E-16, 1.000000000000000000 ) ) ;
#15129=EDGE_CURVE ( 'NONE', #1903, #12174, #29737, .T. ) ;
#15134=ORIENTED_EDGE ( 'NONE', *, *, #15690, .T. ) ;
#15138=CARTESIAN_POINT ( 'NONE',  ( -5.069257791428325888, 7.538175180318473778, 13.22130136205108819 ) ) ;
#15149=CARTESIAN_POINT ( 'NONE',  ( -0.1262659238204836554, -8.999114229549588728, 21.50000000000000000 ) ) ;
#15161=ORIENTED_EDGE ( 'NONE', *, *, #17564, .T. ) ;
#15165=DIRECTION ( 'NONE',  ( 0.000000000000000000, 0.000000000000000000, 1.000000000000000000 ) ) ;
#15169=DIRECTION ( 'NONE',  ( 1.000000000000000000, 0.000000000000000000, 0.000000000000000000 ) ) ;
#15188=CARTESIAN_POINT ( 'NONE',  ( -7.663215745754974328, 3.196529495465474380, -1.500000000000001332 ) ) ;
#15189=ORIENTED_EDGE ( 'NONE', *, *, #24608, .T. ) ;
#15190=PLANE ( 'NONE',  #29732 ) ;
#15199=AXIS2_PLACEMENT_3D ( 'NONE', #7652, #767, #26674 ) ;
#15206=DIRECTION ( 'NONE',  ( 0.000000000000000000, -1.132880637372608986E-16, 1.000000000000000000 ) ) ;
#15234=LINE ( 'NONE', #29611, #7123 ) ;
#15242=ORIENTED_EDGE ( 'NONE', *, *, #12798, .F. ) ;
#15250=CARTESIAN_POINT ( 'NONE',  ( 0.6237340761795171495, -8.999114229549588728, 21.50000000000000000 ) ) ;
#15259=VECTOR ( 'NONE', #19994, 1000.000000000000000 ) ;
#15275=CIRCLE ( 'NONE', #28216, 0.7500000000000004441 ) ;
#15288=ORIENTED_EDGE ( 'NONE', *, *, #16452, .T. ) ;
#15290=VECTOR ( 'NONE', #18452, 1000.000000000000000 ) ;
#15298=DIRECTION ( 'NONE',  ( 0.000000000000000000, 0.000000000000000000, 1.000000000000000000 ) ) ;
#15315=EDGE_CURVE ( 'NONE', #16202, #3179, #11292, .T. ) ;
#15320=DIRECTION ( 'NONE',  ( 1.000000000000000000, 0.000000000000000000, -0.000000000000000000 ) ) ;
#15324=LINE ( 'NONE', #3025, #18276 ) ;
#15325=DIRECTION ( 'NONE',  ( 1.000000000000000000, 0.000000000000000000, -0.000000000000000000 ) ) ;
#15336=CARTESIAN_POINT ( 'NONE',  ( -8.499586724479453181, -2.959227181723774525, 21.50000000000000000 ) ) ;
#15340=CARTESIAN_POINT ( 'NONE',  ( -8.090471615930056259, 1.687027447297517080, 21.50000000000000000 ) ) ;
#15374=ORIENTED_EDGE ( 'NONE', *, *, #24817, .T. ) ;
#15377=DIRECTION ( 'NONE',  ( 0.000000000000000000, 1.000000000000000000, 0.000000000000000000 ) ) ;
#15386=AXIS2_PLACEMENT_3D ( 'NONE', #10460, #3441, #14467 ) ;
#15388=CARTESIAN_POINT ( 'NONE',  ( -8.999114229549592281, 0.1262659238205133538, 21.50000000000000000 ) ) ;
#15397=ORIENTED_EDGE ( 'NONE', *, *, #22763, .T. ) ;
#15400=ORIENTED_EDGE ( 'NONE', *, *, #10380, .T. ) ;
#15419=CARTESIAN_POINT ( 'NONE',  ( -7.106594496258223259, -4.390207617113929039, -1.500000000000002220 ) ) ;
#15425=VERTEX_POINT ( 'NONE', #18771 ) ;
#15444=DIRECTION ( 'NONE',  ( 0.000000000000000000, -1.132880637372608986E-16, 1.000000000000000000 ) ) ;
#15449=EDGE_CURVE ( 'NONE', #6070, #9872, #23431, .T. ) ;
#15452=CIRCLE ( 'NONE', #2998, 9.084132297865673777 ) ;
#15469=DIRECTION ( 'NONE',  ( 0.000000000000000000, -1.132880637372608986E-16, 1.000000000000000000 ) ) ;
#15476=ORIENTED_EDGE ( 'NONE', *, *, #26618, .T. ) ;
#15487=CARTESIAN_POINT ( 'NONE',  ( -5.131244434206278626, -6.812559277181949646, -1.500000000000002665 ) ) ;
#15499=CARTESIAN_POINT ( 'NONE',  ( -8.999114229549592281, 0.1262659238205133538, 21.50000000000000000 ) ) ;
#15519=DIRECTION ( 'NONE',  ( 1.000000000000000000, 0.000000000000000000, 0.000000000000000000 ) ) ;
#15526=DIRECTION ( 'NONE',  ( 0.000000000000000000, 1.132880637372608986E-16, -1.000000000000000000 ) ) ;
#15529=LINE ( 'NONE', #20056, #19227 ) ;
#15532=DIRECTION ( 'NONE',  ( 1.000000000000000000, 0.000000000000000000, 0.000000000000000000 ) ) ;
#15534=AXIS2_PLACEMENT_3D ( 'NONE', #6906, #14213, #16260 ) ;
#15535=CARTESIAN_POINT ( 'NONE',  ( -0.8762659238204844048, -8.999114229549588728, 21.50000000000000000 ) ) ;
#15539=EDGE_LOOP ( 'NONE', ( #1197, #16089, #5210 ) ) ;
#15542=FACE_OUTER_BOUND ( 'NONE', #3664, .T. ) ;
#15544=AXIS2_PLACEMENT_3D ( 'NONE', #1830, #9010, #11355 ) ;
#15556=ORIENTED_EDGE ( 'NONE', *, *, #25410, .T. ) ;
#15557=AXIS2_PLACEMENT_3D ( 'NONE', #18922, #6601, #14063 ) ;
#15560=VERTEX_POINT ( 'NONE', #19963 ) ;
#15566=DIRECTION ( 'NONE',  ( -0.000000000000000000, 1.132880637372608986E-16, -1.000000000000000000 ) ) ;
#15591=ORIENTED_EDGE ( 'NONE', *, *, #28196, .F. ) ;
#15594=VERTEX_POINT ( 'NONE', #26839 ) ;
#15595=CIRCLE ( 'NONE', #3138, 0.7499999999999988898 ) ;
#15600=ORIENTED_EDGE ( 'NONE', *, *, #26727, .F. ) ;
#15605=CARTESIAN_POINT ( 'NONE',  ( 7.488956955540400529, 5.141690706682902068, -1.500000000000001110 ) ) ;
#15615=CIRCLE ( 'NONE', #2166, 0.7500000000000006661 ) ;
#15625=DIRECTION ( 'NONE',  ( 0.000000000000000000, 1.000000000000000000, 0.000000000000000000 ) ) ;
#15632=VERTEX_POINT ( 'NONE', #5622 ) ;
#15656=EDGE_CURVE ( 'NONE', #6824, #6045, #7198, .T. ) ;
#15663=EDGE_CURVE ( 'NONE', #27328, #1692, #29791, .T. ) ;
#15679=DIRECTION ( 'NONE',  ( 0.000000000000000000, 1.000000000000000000, 1.132880637372608986E-16 ) ) ;
#15685=CARTESIAN_POINT ( 'NONE',  ( -5.141690706682823020, 7.488956955540454707, -1.500000000000000888 ) ) ;
#15690=EDGE_CURVE ( 'NONE', #6045, #28904, #25100, .T. ) ;
#15692=EDGE_CURVE ( 'NONE', #25420, #4539, #13568, .T. ) ;
#15694=FACE_OUTER_BOUND ( 'NONE', #5819, .T. ) ;
#15695=EDGE_CURVE ( 'NONE', #29091, #8467, #19637, .T. ) ;
#15696=DIRECTION ( 'NONE',  ( 1.000000000000000000, 0.000000000000000000, -0.000000000000000000 ) ) ;
#15711=EDGE_LOOP ( 'NONE', ( #25554, #7156 ) ) ;
#15718=FACE_OUTER_BOUND ( 'NONE', #10936, .T. ) ;
#15721=ORIENTED_EDGE ( 'NONE', *, *, #1983, .T. ) ;
#15737=ORIENTED_EDGE ( 'NONE', *, *, #19894, .F. ) ;
#15738=DIRECTION ( 'NONE',  ( 1.000000000000000000, 0.000000000000000000, -0.000000000000000000 ) ) ;
#15740=PLANE ( 'NONE',  #16968 ) ;
#15741=ORIENTED_EDGE ( 'NONE', *, *, #16800, .T. ) ;
#15766=VERTEX_POINT ( 'NONE', #11213 ) ;
#15794=VECTOR ( 'NONE', #1337, 1000.000000000000000 ) ;
#15805=EDGE_CURVE ( 'NONE', #25108, #11004, #22136, .T. ) ;
#15807=AXIS2_PLACEMENT_3D ( 'NONE', #21386, #2054, #14057 ) ;
#15810=ORIENTED_EDGE ( 'NONE', *, *, #29867, .F. ) ;
#15826=VERTEX_POINT ( 'NONE', #23656 ) ;
#15835=ADVANCED_FACE ( 'NONE', ( #120 ), #28517, .F. ) ;
#15841=CIRCLE ( 'NONE', #27815, 9.084132297865673777 ) ;
#15845=FACE_OUTER_BOUND ( 'NONE', #20453, .T. ) ;
#15853=CIRCLE ( 'NONE', #28305, 0.7500000000000006661 ) ;
#15858=LINE ( 'NONE', #20386, #12913 ) ;
#15860=VECTOR ( 'NONE', #19827, 1000.000000000000000 ) ;
#15873=CYLINDRICAL_SURFACE ( 'NONE', #16040, 0.7500000000000006661 ) ;
#15897=ORIENTED_EDGE ( 'NONE', *, *, #13799, .T. ) ;
#15905=CARTESIAN_POINT ( 'NONE',  ( 8.817355867515813017, 2.185336383880231992, -1.500000000000001554 ) ) ;
#15910=AXIS2_PLACEMENT_3D ( 'NONE', #11479, #30487, #4747 ) ;
#15925=EDGE_LOOP ( 'NONE', ( #10517, #5773, #22669, #6411 ) ) ;
#15934=EDGE_LOOP ( 'NONE', ( #30643, #27243, #2464, #10034 ) ) ;
#15940=CARTESIAN_POINT ( 'NONE',  ( 1.492780340587499928E-15, -12.18947652193949693, 29.43090101791767665 ) ) ;
#15950=DIRECTION ( 'NONE',  ( 1.000000000000000000, 0.000000000000000000, 0.000000000000000000 ) ) ;
#15951=VERTEX_POINT ( 'NONE', #12292 ) ;
#15954=ORIENTED_EDGE ( 'NONE', *, *, #3911, .T. ) ;
#15958=DIRECTION ( 'NONE',  ( 0.000000000000000000, 1.132880637372608986E-16, -1.000000000000000000 ) ) ;
#15959=CYLINDRICAL_SURFACE ( 'NONE', #8784, 0.7500000000000015543 ) ;
#15963=ORIENTED_EDGE ( 'NONE', *, *, #10532, .T. ) ;
#15965=CIRCLE ( 'NONE', #24871, 0.7499999999999997780 ) ;
#15975=EDGE_LOOP ( 'NONE', ( #23245, #25053, #1496, #7077 ) ) ;
#15979=CARTESIAN_POINT ( 'NONE',  ( -4.608906612435655248, -7.730328572437724866, 21.50000000000000000 ) ) ;
#15987=DIRECTION ( 'NONE',  ( 0.000000000000000000, -1.132880637372608986E-16, 1.000000000000000000 ) ) ;
#15989=ORIENTED_EDGE ( 'NONE', *, *, #4389, .T. ) ;
#16010=DIRECTION ( 'NONE',  ( 0.000000000000000000, 0.000000000000000000, 1.000000000000000000 ) ) ;
#16011=CARTESIAN_POINT ( 'NONE',  ( -7.392982946727046034, 5.278755796068742789, 13.22130136205108819 ) ) ;
#16013=EDGE_LOOP ( 'NONE', ( #6376, #24548, #11163, #20879 ) ) ;
#16022=ADVANCED_FACE ( 'NONE', ( #9002 ), #13220, .F. ) ;
#16023=DIRECTION ( 'NONE',  ( -0.000000000000000000, -0.000000000000000000, 1.000000000000000000 ) ) ;
#16026=DIRECTION ( 'NONE',  ( 0.000000000000000000, 0.000000000000000000, 1.000000000000000000 ) ) ;
#16031=ADVANCED_FACE ( 'NONE', ( #27565 ), #22708, .F. ) ;
#16035=CARTESIAN_POINT ( 'NONE',  ( 0.000000000000000000, 1.699320956058915452E-16, -1.500000000000001776 ) ) ;
#16036=CARTESIAN_POINT ( 'NONE',  ( 0.6210184355499436260, -9.062880100047301823, 13.22130136205108641 ) ) ;
#16040=AXIS2_PLACEMENT_3D ( 'NONE', #2128, #16023, #25392 ) ;
#16043=VERTEX_POINT ( 'NONE', #18515 ) ;
#16047=CARTESIAN_POINT ( 'NONE',  ( 0.000000000000000000, 1.699320956058915452E-16, -1.500000000000001776 ) ) ;
#16051=AXIS2_PLACEMENT_3D ( 'NONE', #17615, #8106, #21696 ) ;
#16052=CARTESIAN_POINT ( 'NONE',  ( 1.687027447297431371, 8.840471615930075799, 21.50000000000000000 ) ) ;
#16054=DIRECTION ( 'NONE',  ( -0.000000000000000000, 1.132880637372608986E-16, -1.000000000000000000 ) ) ;
#16055=ORIENTED_EDGE ( 'NONE', *, *, #16402, .F. ) ;
#16058=CARTESIAN_POINT ( 'NONE',  ( -7.341751895053199917, 5.349779314757666882, 21.50000000000000000 ) ) ;
#16063=EDGE_CURVE ( 'NONE', #9274, #28044, #6502, .T. ) ;
#16067=EDGE_CURVE ( 'NONE', #6047, #24171, #9689, .T. ) ;
#16071=CARTESIAN_POINT ( 'NONE',  ( 2.959227181723801170, -8.499586724479446076, -3.621320343559650379 ) ) ;
#16087=EDGE_CURVE ( 'NONE', #14124, #26044, #2737, .T. ) ;
#16089=ORIENTED_EDGE ( 'NONE', *, *, #9397, .F. ) ;
#16120=EDGE_CURVE ( 'NONE', #23454, #8444, #7890, .T. ) ;
#16126=FACE_BOUND ( 'NONE', #27421, .T. ) ;
#16130=CARTESIAN_POINT ( 'NONE',  ( -6.980328572437709767, 4.608906612435681005, -1.500000000000001332 ) ) ;
#16153=DIRECTION ( 'NONE',  ( 0.000000000000000000, 1.000000000000000000, 0.000000000000000000 ) ) ;
#16158=AXIS2_PLACEMENT_3D ( 'NONE', #17942, #20873, #16194 ) ;
#16160=DIRECTION ( 'NONE',  ( 0.000000000000000000, 0.000000000000000000, 1.000000000000000000 ) ) ;
#16168=DIRECTION ( 'NONE',  ( 0.000000000000000000, -1.132880637372608986E-16, 1.000000000000000000 ) ) ;
#16177=FACE_OUTER_BOUND ( 'NONE', #11541, .T. ) ;
#16190=LINE ( 'NONE', #4956, #16593 ) ;
#16191=ADVANCED_FACE ( 'NONE', ( #14897 ), #396, .F. ) ;
#16194=DIRECTION ( 'NONE',  ( 0.000000000000000000, 1.000000000000000000, 0.000000000000000000 ) ) ;
#16202=VERTEX_POINT ( 'NONE', #15188 ) ;
#16211=CARTESIAN_POINT ( 'NONE',  ( -0.1262659238204836554, -8.999114229549588728, -1.500000000000002665 ) ) ;
#16220=EDGE_LOOP ( 'NONE', ( #3314, #15810, #8662, #6913 ) ) ;
#16247=DIRECTION ( 'NONE',  ( 0.000000000000000000, 1.000000000000000000, 1.193512090021232842E-16 ) ) ;
#16260=DIRECTION ( 'NONE',  ( 1.000000000000000000, 0.000000000000000000, -0.000000000000000000 ) ) ;
#16268=VERTEX_POINT ( 'NONE', #13031 ) ;
#16274=ORIENTED_EDGE ( 'NONE', *, *, #16067, .T. ) ;
#16293=LINE ( 'NONE', #25510, #5810 ) ;
#16300=CARTESIAN_POINT ( 'NONE',  ( 9.041888939645136958, -0.8750451464062836138, 13.22130136205108819 ) ) ;
#16329=DIRECTION ( 'NONE',  ( 0.000000000000000000, 1.000000000000000000, 0.000000000000000000 ) ) ;
#16367=AXIS2_PLACEMENT_3D ( 'NONE', #18396, #13247, #11052 ) ;
#16368=VERTEX_POINT ( 'NONE', #16130 ) ;
#16369=DIRECTION ( 'NONE',  ( 0.000000000000000000, 1.000000000000000000, 1.193512090021232842E-16 ) ) ;
#16371=DIRECTION ( 'NONE',  ( 0.000000000000000000, 1.132880637372608986E-16, -1.000000000000000000 ) ) ;
#16374=ORIENTED_EDGE ( 'NONE', *, *, #13979, .F. ) ;
#16376=DIRECTION ( 'NONE',  ( 1.000000000000000000, 0.000000000000000000, 0.000000000000000000 ) ) ;
#16394=DIRECTION ( 'NONE',  ( -0.000000000000000000, -0.000000000000000000, 1.000000000000000000 ) ) ;
#16402=EDGE_CURVE ( 'NONE', #26020, #11549, #11214, .T. ) ;
#16406=DIRECTION ( 'NONE',  ( 1.000000000000000000, 0.000000000000000000, 0.000000000000000000 ) ) ;
#16415=DIRECTION ( 'NONE',  ( 0.000000000000000000, -1.132880637372608986E-16, 1.000000000000000000 ) ) ;
#16417=DIRECTION ( 'NONE',  ( -0.000000000000000000, 1.132880637372608986E-16, -1.000000000000000000 ) ) ;
#16424=ORIENTED_EDGE ( 'NONE', *, *, #8311, .T. ) ;
#16433=ORIENTED_EDGE ( 'NONE', *, *, #4203, .T. ) ;
#16452=EDGE_CURVE ( 'NONE', #5107, #22385, #662, .T. ) ;
#16464=DIRECTION ( 'NONE',  ( 0.000000000000000000, 0.000000000000000000, 1.000000000000000000 ) ) ;
#16483=AXIS2_PLACEMENT_3D ( 'NONE', #18177, #27683, #6311 ) ;
#16487=DIRECTION ( 'NONE',  ( -0.000000000000000000, -0.000000000000000000, 1.000000000000000000 ) ) ;
#16495=ORIENTED_EDGE ( 'NONE', *, *, #28412, .F. ) ;
#16497=CARTESIAN_POINT ( 'NONE',  ( -8.249114229549590505, 0.1262659238205133538, 21.50000000000000000 ) ) ;
#16506=ORIENTED_EDGE ( 'NONE', *, *, #2539, .F. ) ;
#16517=AXIS2_PLACEMENT_3D ( 'NONE', #101, #4769, #23795 ) ;
#16526=DIRECTION ( 'NONE',  ( 0.000000000000000000, 0.000000000000000000, 1.000000000000000000 ) ) ;
#16533=CARTESIAN_POINT ( 'NONE',  ( -6.482337650448453559, -6.364020599487773211, 21.50000000000000000 ) ) ;
#16535=VERTEX_POINT ( 'NONE', #16897 ) ;
#16536=AXIS2_PLACEMENT_3D ( 'NONE', #2865, #22353, #17367 ) ;
#16541=DIRECTION ( 'NONE',  ( 0.000000000000000000, 1.000000000000000000, 1.193512090021232842E-16 ) ) ;
#16561=CARTESIAN_POINT ( 'NONE',  ( 0.000000000000000000, 0.000000000000000000, -87.50000000000000000 ) ) ;
#16564=DIRECTION ( 'NONE',  ( 0.000000000000000000, -1.132880637372608986E-16, 1.000000000000000000 ) ) ;
#16567=DIRECTION ( 'NONE',  ( 0.000000000000000000, -1.132880637372608986E-16, 1.000000000000000000 ) ) ;
#16573=DIRECTION ( 'NONE',  ( 1.000000000000000000, 0.000000000000000000, 0.000000000000000000 ) ) ;
#16587=EDGE_CURVE ( 'NONE', #7713, #14972, #23657, .T. ) ;
#16593=VECTOR ( 'NONE', #14008, 1000.000000000000000 ) ;
#16597=VERTEX_POINT ( 'NONE', #25138 ) ;
#16598=CIRCLE ( 'NONE', #3162, 9.084132297865673777 ) ;
#16606=AXIS2_PLACEMENT_3D ( 'NONE', #30463, #30772, #23134 ) ;
#16609=DIRECTION ( 'NONE',  ( 1.000000000000000000, 0.000000000000000000, -0.000000000000000000 ) ) ;
#16615=CARTESIAN_POINT ( 'NONE',  ( 0.1262659238204208167, 8.999114229549594057, -1.500000000000000888 ) ) ;
#16625=ADVANCED_FACE ( 'NONE', ( #3478 ), #20317, .T. ) ;
#16638=CARTESIAN_POINT ( 'NONE',  ( 7.341751895053238108, -5.349779314757616255, -1.500000000000002442 ) ) ;
#16649=DIRECTION ( 'NONE',  ( -0.000000000000000000, 1.132880637372608986E-16, -1.000000000000000000 ) ) ;
#16652=EDGE_CURVE ( 'NONE', #15594, #27497, #23154, .T. ) ;
#16686=ORIENTED_EDGE ( 'NONE', *, *, #16587, .F. ) ;
#16708=CARTESIAN_POINT ( 'NONE',  ( -8.499586724479453181, -2.959227181723774525, 21.50000000000000000 ) ) ;
#16717=CIRCLE ( 'NONE', #3269, 0.7499999999999993339 ) ;
#16740=DIRECTION ( 'NONE',  ( 1.000000000000000000, 0.000000000000000000, 0.000000000000000000 ) ) ;
#16742=ORIENTED_EDGE ( 'NONE', *, *, #9043, .T. ) ;
#16744=EDGE_CURVE ( 'NONE', #20718, #6357, #18213, .T. ) ;
#16748=ORIENTED_EDGE ( 'NONE', *, *, #8241, .F. ) ;
#16749=CIRCLE ( 'NONE', #28716, 0.7500000000000006661 ) ;
#16756=DIRECTION ( 'NONE',  ( -0.000000000000000000, -0.000000000000000000, 1.000000000000000000 ) ) ;
#16766=CARTESIAN_POINT ( 'NONE',  ( 5.349779314757592275, 7.341751895053254096, 13.22130136205108819 ) ) ;
#16780=DIRECTION ( 'NONE',  ( 0.000000000000000000, 1.000000000000000000, 1.193512090021232842E-16 ) ) ;
#16781=EDGE_CURVE ( 'NONE', #5107, #8541, #24676, .T. ) ;
#16791=EDGE_CURVE ( 'NONE', #28030, #22385, #24154, .T. ) ;
#16798=LINE ( 'NONE', #419, #3434 ) ;
#16800=EDGE_CURVE ( 'NONE', #386, #5107, #10724, .T. ) ;
#16802=DIRECTION ( 'NONE',  ( -0.000000000000000000, -0.000000000000000000, 1.000000000000000000 ) ) ;
#16811=ORIENTED_EDGE ( 'NONE', *, *, #11617, .T. ) ;
#16832=CIRCLE ( 'NONE', #4381, 0.7499999999999997780 ) ;
#16836=DIRECTION ( 'NONE',  ( 0.000000000000000000, 1.132880637372608986E-16, -1.000000000000000000 ) ) ;
#16841=CARTESIAN_POINT ( 'NONE',  ( -8.159193615868369776, 3.993622308618967498, 13.22130136205108819 ) ) ;
#16856=ADVANCED_FACE ( 'NONE', ( #21516 ), #475, .F. ) ;
#16857=DIRECTION ( 'NONE',  ( 0.000000000000000000, -1.132880637372608986E-16, 1.000000000000000000 ) ) ;
#16858=CIRCLE ( 'NONE', #22842, 12.18947652193948272 ) ;
#16860=DIRECTION ( 'NONE',  ( 0.000000000000000000, 0.000000000000000000, 1.000000000000000000 ) ) ;
#16866=DIRECTION ( 'NONE',  ( 0.000000000000000000, 1.000000000000000000, 0.000000000000000000 ) ) ;
#16877=AXIS2_PLACEMENT_3D ( 'NONE', #9317, #18842, #28360 ) ;
#16879=CIRCLE ( 'NONE', #10410, 9.084132297865673777 ) ;
#16893=ORIENTED_EDGE ( 'NONE', *, *, #24437, .F. ) ;
#16897=CARTESIAN_POINT ( 'NONE',  ( -3.640207617113898841, 7.856594496258241023, -1.500000000000000888 ) ) ;
#16898=DIRECTION ( 'NONE',  ( 0.000000000000000000, 0.000000000000000000, 1.000000000000000000 ) ) ;
#16900=ORIENTED_EDGE ( 'NONE', *, *, #21022, .F. ) ;
#16905=ORIENTED_EDGE ( 'NONE', *, *, #11258, .T. ) ;
#16908=DIRECTION ( 'NONE',  ( 0.000000000000000000, 1.000000000000000000, 1.193512090021232842E-16 ) ) ;
#16916=DIRECTION ( 'NONE',  ( -0.000000000000000000, -0.000000000000000000, 1.000000000000000000 ) ) ;
#16950=CYLINDRICAL_SURFACE ( 'NONE', #6829, 0.7500000000000006661 ) ;
#16968=AXIS2_PLACEMENT_3D ( 'NONE', #27918, #16054, #25571 ) ;
#16979=CARTESIAN_POINT ( 'NONE',  ( 0.1262659238204208167, 8.999114229549594057, 21.50000000000000000 ) ) ;
#16997=EDGE_CURVE ( 'NONE', #30243, #12174, #23174, .T. ) ;
#17012=ORIENTED_EDGE ( 'NONE', *, *, #16652, .T. ) ;
#17033=CIRCLE ( 'NONE', #23503, 0.7500000000000006661 ) ;
#17047=VERTEX_POINT ( 'NONE', #2905 ) ;
#17061=EDGE_CURVE ( 'NONE', #17300, #15425, #12258, .T. ) ;
#17063=DIRECTION ( 'NONE',  ( -0.000000000000000000, -0.000000000000000000, 1.000000000000000000 ) ) ;
#17070=VECTOR ( 'NONE', #20522, 1000.000000000000000 ) ;
#17085=DIRECTION ( 'NONE',  ( -0.000000000000000000, 1.132880637372608986E-16, -1.000000000000000000 ) ) ;
#17092=DIRECTION ( 'NONE',  ( 0.000000000000000000, 1.000000000000000000, 0.000000000000000000 ) ) ;
#17097=AXIS2_PLACEMENT_3D ( 'NONE', #7066, #18936, #11597 ) ;
#17104=DIRECTION ( 'NONE',  ( 0.000000000000000000, -1.000000000000000000, -1.132880637372608986E-16 ) ) ;
#17114=CIRCLE ( 'NONE', #9145, 7.500000000000008882 ) ;
#17121=CARTESIAN_POINT ( 'NONE',  ( -6.812559277181930106, 5.881244434206302607, -1.500000000000000888 ) ) ;
#17133=DIRECTION ( 'NONE',  ( 0.000000000000000000, 0.000000000000000000, 1.000000000000000000 ) ) ;
#17145=AXIS2_PLACEMENT_3D ( 'NONE', #23265, #11436, #18003 ) ;
#17156=EDGE_LOOP ( 'NONE', ( #30054, #9172, #16748, #1996 ) ) ;
#17175=EDGE_CURVE ( 'NONE', #15632, #21841, #28738, .T. ) ;
#17182=EDGE_CURVE ( 'NONE', #11519, #5775, #6908, .T. ) ;
#17187=CARTESIAN_POINT ( 'NONE',  ( 8.197313248159948884, -3.914781618004724795, 13.22130136205108819 ) ) ;
#17197=VERTEX_POINT ( 'NONE', #181 ) ;
#17208=AXIS2_PLACEMENT_3D ( 'NONE', #25853, #8864, #13698 ) ;
#17211=CARTESIAN_POINT ( 'NONE',  ( 9.041888939645136958, -0.8750451464062836138, -1.500000000000001776 ) ) ;
#17220=VECTOR ( 'NONE', #17085, 1000.000000000000000 ) ;
#17227=ORIENTED_EDGE ( 'NONE', *, *, #24059, .F. ) ;
#17230=CYLINDRICAL_SURFACE ( 'NONE', #18421, 0.7500000000000006661 ) ;
#17240=CARTESIAN_POINT ( 'NONE',  ( -9.062880100047301823, -0.6210184355499139830, 13.22130136205108819 ) ) ;
#17262=DIRECTION ( 'NONE',  ( 0.000000000000000000, 0.000000000000000000, 1.000000000000000000 ) ) ;
#17284=ORIENTED_EDGE ( 'NONE', *, *, #24101, .T. ) ;
#17292=CARTESIAN_POINT ( 'NONE',  ( 8.413215745754998309, -3.196529495465417980, -1.500000000000002220 ) ) ;
#17300=VERTEX_POINT ( 'NONE', #24188 ) ;
#17301=ORIENTED_EDGE ( 'NONE', *, *, #19964, .T. ) ;
#17307=CIRCLE ( 'NONE', #29761, 9.084132297865673777 ) ;
#17316=ORIENTED_EDGE ( 'NONE', *, *, #24437, .T. ) ;
#17321=AXIS2_PLACEMENT_3D ( 'NONE', #23490, #1679, #23637 ) ;
#17363=ORIENTED_EDGE ( 'NONE', *, *, #4081, .F. ) ;
#17364=CARTESIAN_POINT ( 'NONE',  ( 2.270234684139677217, -8.795879380940574421, 13.22130136205108641 ) ) ;
#17365=PRODUCT_DEFINITION_FORMATION_WITH_SPECIFIED_SOURCE ( 'ANY', '', #4430, .NOT_KNOWN. ) ;
#17367=DIRECTION ( 'NONE',  ( 0.000000000000000000, 1.000000000000000000, 0.000000000000000000 ) ) ;
#17378=CARTESIAN_POINT ( 'NONE',  ( -5.881244434206279514, -6.812559277181949646, -1.500000000000002665 ) ) ;
#17391=EDGE_CURVE ( 'NONE', #3254, #26855, #9251, .T. ) ;
#17393=EDGE_CURVE ( 'NONE', #10427, #28059, #26185, .T. ) ;
#17395=ORIENTED_EDGE ( 'NONE', *, *, #26562, .F. ) ;
#17398=PLANE ( 'NONE',  #19395 ) ;
#17399=VECTOR ( 'NONE', #16756, 1000.000000000000000 ) ;
#17401=DIRECTION ( 'NONE',  ( 0.000000000000000000, -1.132880637372608986E-16, 1.000000000000000000 ) ) ;
#17426=EDGE_CURVE ( 'NONE', #30256, #549, #275, .T. ) ;
#17430=ORIENTED_EDGE ( 'NONE', *, *, #8311, .F. ) ;
#17444=ORIENTED_EDGE ( 'NONE', *, *, #26840, .F. ) ;
#17448=CARTESIAN_POINT ( 'NONE',  ( 7.730328572437743517, -4.608906612435629491, -1.500000000000002220 ) ) ;
#17465=EDGE_LOOP ( 'NONE', ( #13422, #14431, #23140, #17284 ) ) ;
#17470=VERTEX_POINT ( 'NONE', #3614 ) ;
#17472=CIRCLE ( 'NONE', #24945, 9.084132297865673777 ) ;
#17483=CARTESIAN_POINT ( 'NONE',  ( 6.974883619896790954, 5.687793815610376669, -3.621320343559650379 ) ) ;
#17484=DIRECTION ( 'NONE',  ( 0.000000000000000000, 0.000000000000000000, 1.000000000000000000 ) ) ;
#17485=ORIENTED_EDGE ( 'NONE', *, *, #823, .F. ) ;
#17487=VECTOR ( 'NONE', #30590, 1000.000000000000000 ) ;
#17491=CIRCLE ( 'NONE', #19999, 9.084132297865673777 ) ;
#17511=CARTESIAN_POINT ( 'NONE',  ( -8.499586724479453181, -2.959227181723774525, 21.50000000000000000 ) ) ;
#17513=DIRECTION ( 'NONE',  ( 1.000000000000000000, 0.000000000000000000, 0.000000000000000000 ) ) ;
#17517=ORIENTED_EDGE ( 'NONE', *, *, #29772, .F. ) ;
#17518=DIRECTION ( 'NONE',  ( 0.000000000000000000, 1.000000000000000000, 0.000000000000000000 ) ) ;
#17528=CARTESIAN_POINT ( 'NONE',  ( 0.1262659238204208167, 8.999114229549594057, -3.621320343559650379 ) ) ;
#17550=EDGE_LOOP ( 'NONE', ( #18420, #25924 ) ) ;
#17557=EDGE_CURVE ( 'NONE', #11562, #5756, #14837, .T. ) ;
#17564=EDGE_CURVE ( 'NONE', #22385, #20718, #20223, .T. ) ;
#17580=EDGE_CURVE ( 'NONE', #2431, #15951, #9056, .T. ) ;
#17613=EDGE_CURVE ( 'NONE', #11152, #14718, #25212, .T. ) ;
#17615=CARTESIAN_POINT ( 'NONE',  ( -8.884323311075783991, -1.438332125858144295, 21.50000000000000000 ) ) ;
#17616=ORIENTED_EDGE ( 'NONE', *, *, #8241, .T. ) ;
#17647=VERTEX_POINT ( 'NONE', #11695 ) ;
#17653=VECTOR ( 'NONE', #27452, 1000.000000000000000 ) ;
#17655=CARTESIAN_POINT ( 'NONE',  ( 0.000000000000000000, -2.322405306613848348E-14, 117.5000000000000000 ) ) ;
#17665=ORIENTED_EDGE ( 'NONE', *, *, #11878, .F. ) ;
#17666=CARTESIAN_POINT ( 'NONE',  ( -9.033033306777449312, 0.9621688436940326605, 13.22130136205108819 ) ) ;
#17668=EDGE_CURVE ( 'NONE', #14218, #27309, #26708, .T. ) ;
#17700=CARTESIAN_POINT ( 'NONE',  ( -2.209227181723746103, 8.499586724479465616, 21.50000000000000000 ) ) ;
#17705=DIRECTION ( 'NONE',  ( 0.000000000000000000, 0.000000000000000000, 1.000000000000000000 ) ) ;
#17711=DIRECTION ( 'NONE',  ( 0.000000000000000000, 0.000000000000000000, 1.000000000000000000 ) ) ;
#17715=DIRECTION ( 'NONE',  ( -0.000000000000000000, -0.000000000000000000, 1.000000000000000000 ) ) ;
#17720=ORIENTED_EDGE ( 'NONE', *, *, #25240, .T. ) ;
#17723=CARTESIAN_POINT ( 'NONE',  ( -2.270234684139619041, 8.795879380940583303, 13.22130136205108997 ) ) ;
#17731=EDGE_LOOP ( 'NONE', ( #18638, #22772, #8525 ) ) ;
#17740=EDGE_CURVE ( 'NONE', #20169, #7139, #19238, .T. ) ;
#17741=CIRCLE ( 'NONE', #10254, 9.084132297865673777 ) ;
#17742=VERTEX_POINT ( 'NONE', #5753 ) ;
#17746=ORIENTED_EDGE ( 'NONE', *, *, #5907, .T. ) ;
#17752=FACE_OUTER_BOUND ( 'NONE', #25127, .T. ) ;
#17756=EDGE_CURVE ( 'NONE', #12360, #18098, #28712, .T. ) ;
#17760=CIRCLE ( 'NONE', #4304, 9.084132297865673777 ) ;
#17801=CARTESIAN_POINT ( 'NONE',  ( 0.000000000000000000, -2.775557561562891351E-14, 157.4999999999999716 ) ) ;
#17813=CARTESIAN_POINT ( 'NONE',  ( 0.000000000000000000, 7.500000000000000000, -16.50000000000000000 ) ) ;
#17820=CARTESIAN_POINT ( 'NONE',  ( 3.914781618004695041, 8.197313248159959542, 13.22130136205108997 ) ) ;
#17825=AXIS2_PLACEMENT_3D ( 'NONE', #14596, #19431, #26927 ) ;
#17859=ORIENTED_EDGE ( 'NONE', *, *, #23506, .F. ) ;
#17864=CARTESIAN_POINT ( 'NONE',  ( 0.000000000000000000, -2.435693370351110282E-15, 21.50000000000000355 ) ) ;
#17876=VERTEX_POINT ( 'NONE', #5259 ) ;
#17881=CARTESIAN_POINT ( 'NONE',  ( -3.196529495465446402, -8.413215745754985875, 21.50000000000000000 ) ) ;
#17882=ORIENTED_EDGE ( 'NONE', *, *, #8221, .T. ) ;
#17890=DIRECTION ( 'NONE',  ( 0.000000000000000000, 1.132880637372608986E-16, -1.000000000000000000 ) ) ;
#17891=DIRECTION ( 'NONE',  ( -0.000000000000000000, 1.132880637372608986E-16, -1.000000000000000000 ) ) ;
#17894=CARTESIAN_POINT ( 'NONE',  ( 0.8762659238204211221, 8.999114229549594057, 21.50000000000000000 ) ) ;
#17898=ORIENTED_EDGE ( 'NONE', *, *, #28250, .T. ) ;
#17901=CARTESIAN_POINT ( 'NONE',  ( -7.856594496258223259, -4.390207617113929039, 21.50000000000000000 ) ) ;
#17909=AXIS2_PLACEMENT_3D ( 'NONE', #2691, #12201, #21701 ) ;
#17912=DIRECTION ( 'NONE',  ( 1.000000000000000000, 0.000000000000000000, 0.000000000000000000 ) ) ;
#17930=AXIS2_PLACEMENT_3D ( 'NONE', #11426, #25620, #30288 ) ;
#17936=DIRECTION ( 'NONE',  ( 1.000000000000000000, 0.000000000000000000, 0.000000000000000000 ) ) ;
#17942=CARTESIAN_POINT ( 'NONE',  ( -3.196529495465446402, -8.413215745754985875, -1.500000000000002665 ) ) ;
#17949=EDGE_LOOP ( 'NONE', ( #26480, #13535, #2494, #18783 ) ) ;
#17988=EDGE_CURVE ( 'NONE', #17047, #15766, #1330, .T. ) ;
#17989=ORIENTED_EDGE ( 'NONE', *, *, #21561, .F. ) ;
#17994=ORIENTED_EDGE ( 'NONE', *, *, #19172, .F. ) ;
#18003=DIRECTION ( 'NONE',  ( 0.000000000000000000, 1.000000000000000000, 0.000000000000000000 ) ) ;
#18015=VERTEX_POINT ( 'NONE', #20064 ) ;
#18018=DIRECTION ( 'NONE',  ( 0.000000000000000000, -1.000000000000000000, -1.132880637372608986E-16 ) ) ;
#18026=EDGE_LOOP ( 'NONE', ( #8839, #14059, #28527, #13233 ) ) ;
#18030=CIRCLE ( 'NONE', #21479, 0.7500000000000002220 ) ;
#18043=ORIENTED_EDGE ( 'NONE', *, *, #2031, .T. ) ;
#18047=DIRECTION ( 'NONE',  ( 0.000000000000000000, 0.000000000000000000, 1.000000000000000000 ) ) ;
#18055=CARTESIAN_POINT ( 'NONE',  ( 8.795879380940565540, 2.270234684139708303, 21.50000000000000000 ) ) ;
#18060=ORIENTED_EDGE ( 'NONE', *, *, #29510, .F. ) ;
#18062=CARTESIAN_POINT ( 'NONE',  ( 8.817355867515813017, 2.185336383880231992, 21.50000000000000000 ) ) ;
#18067=( LENGTH_UNIT ( ) NAMED_UNIT ( * ) SI_UNIT ( .MILLI., .METRE. ) );
#18082=CIRCLE ( 'NONE', #30508, 0.7500000000000006661 ) ;
#18084=CIRCLE ( 'NONE', #27055, 12.50000000000000000 ) ;
#18091=CARTESIAN_POINT ( 'NONE',  ( -1.687027447297492211, -8.840471615930066918, 21.50000000000000000 ) ) ;
#18094=ORIENTED_EDGE ( 'NONE', *, *, #1521, .F. ) ;
#18095=DIRECTION ( 'NONE',  ( 0.000000000000000000, -1.132880637372608986E-16, 1.000000000000000000 ) ) ;
#18097=ORIENTED_EDGE ( 'NONE', *, *, #14003, .F. ) ;
#18098=VERTEX_POINT ( 'NONE', #8683 ) ;
#18115=VERTEX_POINT ( 'NONE', #17894 ) ;
#18134=VERTEX_POINT ( 'NONE', #20521 ) ;
#18150=DIRECTION ( 'NONE',  ( -0.000000000000000000, -0.000000000000000000, 1.000000000000000000 ) ) ;
#18177=CARTESIAN_POINT ( 'NONE',  ( 0.000000000000000000, 1.699320956058915452E-16, -1.500000000000001776 ) ) ;
#18181=CARTESIAN_POINT ( 'NONE',  ( 3.763133143576435913, -8.268028093133381162, -1.500000000000002665 ) ) ;
#18182=CARTESIAN_POINT ( 'NONE',  ( 7.488956955540398752, 5.141690706682901180, 13.22130136205108819 ) ) ;
#18183=ORIENTED_EDGE ( 'NONE', *, *, #12059, .T. ) ;
#18185=CARTESIAN_POINT ( 'NONE',  ( 0.000000000000000000, 0.000000000000000000, -87.50000000000000000 ) ) ;
#18191=DIRECTION ( 'NONE',  ( 1.000000000000000000, 0.000000000000000000, 0.000000000000000000 ) ) ;
#18199=ADVANCED_FACE ( 'NONE', ( #22959 ), #8492, .F. ) ;
#18205=EDGE_LOOP ( 'NONE', ( #22835, #7418 ) ) ;
#18213=CIRCLE ( 'NONE', #30159, 0.7500000000000006661 ) ;
#18217=ORIENTED_EDGE ( 'NONE', *, *, #8221, .F. ) ;
#18221=CARTESIAN_POINT ( 'NONE',  ( -6.224883619896829146, -5.687793815610328707, 21.50000000000000000 ) ) ;
#18232=AXIS2_PLACEMENT_3D ( 'NONE', #14386, #5960, #27022 ) ;
#18234=CARTESIAN_POINT ( 'NONE',  ( -0.1262659238204836554, -8.999114229549588728, -3.621320343559650379 ) ) ;
#18243=DIRECTION ( 'NONE',  ( 0.000000000000000000, -1.132880637372608986E-16, 1.000000000000000000 ) ) ;
#18246=DIRECTION ( 'NONE',  ( 1.000000000000000000, 0.000000000000000000, 0.000000000000000000 ) ) ;
#18252=VECTOR ( 'NONE', #25282, 1000.000000000000000 ) ;
#18263=CARTESIAN_POINT ( 'NONE',  ( 0.000000000000000000, 12.18947652193946851, 27.94260272410217638 ) ) ;
#18267=ORIENTED_EDGE ( 'NONE', *, *, #17580, .F. ) ;
#18275=CARTESIAN_POINT ( 'NONE',  ( -6.974883619896829146, -5.687793815610328707, 21.50000000000000000 ) ) ;
#18276=VECTOR ( 'NONE', #24853, 1000.000000000000000 ) ;
#18291=AXIS2_PLACEMENT_3D ( 'NONE', #9092, #8643, #27827 ) ;
#18292=ORIENTED_EDGE ( 'NONE', *, *, #16452, .F. ) ;
#18293=CARTESIAN_POINT ( 'NONE',  ( 9.041888939645136958, -0.8750451464062836138, 21.50000000000000000 ) ) ;
#18296=CARTESIAN_POINT ( 'NONE',  ( -8.499586724479453181, -2.959227181723774525, -3.621320343559650379 ) ) ;
#18303=ORIENTED_EDGE ( 'NONE', *, *, #11135, .T. ) ;
#18314=DIRECTION ( 'NONE',  ( 1.000000000000000000, 0.000000000000000000, 0.000000000000000000 ) ) ;
#18316=EDGE_CURVE ( 'NONE', #13370, #2118, #831, .T. ) ;
#18323=DIRECTION ( 'NONE',  ( 0.000000000000000000, 0.000000000000000000, 1.000000000000000000 ) ) ;
#18324=EDGE_LOOP ( 'NONE', ( #12420, #21618, #26887 ) ) ;
#18335=DIRECTION ( 'NONE',  ( 0.000000000000000000, 1.000000000000000000, 0.000000000000000000 ) ) ;
#18347=AXIS2_PLACEMENT_3D ( 'NONE', #7228, #28607, #16908 ) ;
#18349=CARTESIAN_POINT ( 'NONE',  ( 0.000000000000000000, 0.000000000000000000, -87.50000000000000000 ) ) ;
#18370=EDGE_CURVE ( 'NONE', #1375, #28044, #23237, .T. ) ;
#18378=LINE ( 'NONE', #27727, #27811 ) ;
#18384=CARTESIAN_POINT ( 'NONE',  ( -0.1262659238204836554, -8.999114229549588728, -3.621320343559650379 ) ) ;
#18392=AXIS2_PLACEMENT_3D ( 'NONE', #20206, #17891, #13522 ) ;
#18396=CARTESIAN_POINT ( 'NONE',  ( -4.390207617113899730, 7.856594496258241023, -3.621320343559650379 ) ) ;
#18398=EDGE_CURVE ( 'NONE', #15560, #21169, #6887, .T. ) ;
#18401=CIRCLE ( 'NONE', #3946, 0.7499999999999991118 ) ;
#18413=DIRECTION ( 'NONE',  ( 0.000000000000000000, 1.132880637372608986E-16, -1.000000000000000000 ) ) ;
#18420=ORIENTED_EDGE ( 'NONE', *, *, #24240, .F. ) ;
#18421=AXIS2_PLACEMENT_3D ( 'NONE', #23939, #233, #11953 ) ;
#18422=ORIENTED_EDGE ( 'NONE', *, *, #25781, .F. ) ;
#18423=EDGE_CURVE ( 'NONE', #28337, #18904, #12802, .T. ) ;
#18438=ORIENTED_EDGE ( 'NONE', *, *, #13211, .F. ) ;
#18449=DIRECTION ( 'NONE',  ( -4.625929269271481378E-15, 1.000000000000000000, 0.000000000000000000 ) ) ;
#18452=DIRECTION ( 'NONE',  ( -0.000000000000000000, -0.000000000000000000, 1.000000000000000000 ) ) ;
#18462=CARTESIAN_POINT ( 'NONE',  ( 1.438332125858173605, -8.884323311075778662, -1.500000000000002665 ) ) ;
#18485=ORIENTED_EDGE ( 'NONE', *, *, #17061, .T. ) ;
#18493=LINE ( 'NONE', #20815, #25834 ) ;
#18497=DIRECTION ( 'NONE',  ( 0.000000000000000000, 0.000000000000000000, 1.000000000000000000 ) ) ;
#18509=DIRECTION ( 'NONE',  ( 1.000000000000000000, 0.000000000000000000, 0.000000000000000000 ) ) ;
#18515=CARTESIAN_POINT ( 'NONE',  ( 5.278755796068665518, 7.392982946727100213, -1.500000000000000888 ) ) ;
#18516=ORIENTED_EDGE ( 'NONE', *, *, #19851, .F. ) ;
#18527=ORIENTED_EDGE ( 'NONE', *, *, #26344, .F. ) ;
#18544=ORIENTED_EDGE ( 'NONE', *, *, #24279, .F. ) ;
#18548=DIRECTION ( 'NONE',  ( -0.000000000000000000, -0.000000000000000000, 1.000000000000000000 ) ) ;
#18592=VERTEX_POINT ( 'NONE', #19590 ) ;
#18638=ORIENTED_EDGE ( 'NONE', *, *, #23669, .F. ) ;
#18643=ORIENTED_EDGE ( 'NONE', *, *, #28412, .T. ) ;
#18647=CYLINDRICAL_SURFACE ( 'NONE', #14024, 10.00000000000003375 ) ;
#18653=ORIENTED_EDGE ( 'NONE', *, *, #19693, .T. ) ;
#18656=CARTESIAN_POINT ( 'NONE',  ( 6.482337650448408262, 6.364020599487815844, 13.22130136205108819 ) ) ;
#18666=ORIENTED_EDGE ( 'NONE', *, *, #14683, .T. ) ;
#18671=VECTOR ( 'NONE', #8010, 1000.000000000000000 ) ;
#18683=DIRECTION ( 'NONE',  ( 1.000000000000000000, 0.000000000000000000, -0.000000000000000000 ) ) ;
#18685=EDGE_LOOP ( 'NONE', ( #6985, #7719, #556, #17363 ) ) ;
#18688=ORIENTED_EDGE ( 'NONE', *, *, #20067, .T. ) ;
#18710=DIRECTION ( 'NONE',  ( 0.000000000000000000, -1.132880637372608986E-16, 1.000000000000000000 ) ) ;
#18712=ORIENTED_EDGE ( 'NONE', *, *, #23115, .T. ) ;
#18715=AXIS2_PLACEMENT_3D ( 'NONE', #6076, #5927, #8439 ) ;
#18718=ORIENTED_EDGE ( 'NONE', *, *, #13934, .F. ) ;
#18725=EDGE_CURVE ( 'NONE', #4539, #1968, #23263, .T. ) ;
#18731=EDGE_CURVE ( 'NONE', #1458, #23298, #29107, .T. ) ;
#18746=PLANE ( 'NONE',  #21607 ) ;
#18752=DIRECTION ( 'NONE',  ( -0.000000000000000000, 1.132880637372608986E-16, -1.000000000000000000 ) ) ;
#18761=AXIS2_PLACEMENT_3D ( 'NONE', #19450, #17262, #12129 ) ;
#18767=VECTOR ( 'NONE', #3613, 1000.000000000000000 ) ;
#18771=CARTESIAN_POINT ( 'NONE',  ( -9.062880100047301823, -0.6210184355499139830, -1.500000000000001776 ) ) ;
#18774=EDGE_LOOP ( 'NONE', ( #17227, #18438 ) ) ;
#18777=CARTESIAN_POINT ( 'NONE',  ( -3.914781618004753216, -8.197313248159932897, -1.500000000000002665 ) ) ;
#18783=ORIENTED_EDGE ( 'NONE', *, *, #28430, .F. ) ;
#18810=AXIS2_PLACEMENT_3D ( 'NONE', #25542, #26000, #4628 ) ;
#18814=ORIENTED_EDGE ( 'NONE', *, *, #2750, .F. ) ;
#18821=VECTOR ( 'NONE', #13771, 1000.000000000000000 ) ;
#18828=DIRECTION ( 'NONE',  ( -0.000000000000000000, 1.132880637372608986E-16, -1.000000000000000000 ) ) ;
#18836=DIRECTION ( 'NONE',  ( -0.000000000000000000, -0.000000000000000000, 1.000000000000000000 ) ) ;
#18842=DIRECTION ( 'NONE',  ( -0.000000000000000000, -0.000000000000000000, 1.000000000000000000 ) ) ;
#18849=ORIENTED_EDGE ( 'NONE', *, *, #1790, .F. ) ;
#18852=ORIENTED_EDGE ( 'NONE', *, *, #29443, .F. ) ;
#18865=EDGE_LOOP ( 'NONE', ( #28207, #28678, #11032, #21166 ) ) ;
#18878=DIRECTION ( 'NONE',  ( 1.000000000000000000, 0.000000000000000000, 0.000000000000000000 ) ) ;
#18889=AXIS2_PLACEMENT_3D ( 'NONE', #13673, #13817, #23157 ) ;
#18904=VERTEX_POINT ( 'NONE', #11761 ) ;
#18910=CARTESIAN_POINT ( 'NONE',  ( -8.884323311075783991, -1.438332125858144295, -3.621320343559650379 ) ) ;
#18917=CIRCLE ( 'NONE', #4970, 10.00000000000003730 ) ;
#18922=CARTESIAN_POINT ( 'NONE',  ( -6.812559277181930106, 5.881244434206302607, -3.621320343559650379 ) ) ;
#18936=DIRECTION ( 'NONE',  ( 0.000000000000000000, 1.132880637372608986E-16, -1.000000000000000000 ) ) ;
#18942=AXIS2_PLACEMENT_3D ( 'NONE', #1289, #25139, #17513 ) ;
#18966=ORIENTED_EDGE ( 'NONE', *, *, #17557, .F. ) ;
#18981=ORIENTED_EDGE ( 'NONE', *, *, #11311, .F. ) ;
#18984=CARTESIAN_POINT ( 'NONE',  ( 0.000000000000000000, 1.604273173167211147E-31, -87.50000000000000000 ) ) ;
#18998=DIRECTION ( 'NONE',  ( 1.000000000000000000, 0.000000000000000000, 0.000000000000000000 ) ) ;
#19013=EDGE_CURVE ( 'NONE', #17197, #1665, #14786, .T. ) ;
#19015=ORIENTED_EDGE ( 'NONE', *, *, #3131, .T. ) ;
#19020=AXIS2_PLACEMENT_3D ( 'NONE', #18984, #18828, #17092 ) ;
#19026=CARTESIAN_POINT ( 'NONE',  ( 4.390207617113956573, -7.856594496258208160, 21.50000000000000000 ) ) ;
#19029=ORIENTED_EDGE ( 'NONE', *, *, #3488, .F. ) ;
#19053=CARTESIAN_POINT ( 'NONE',  ( -0.9621688436940065703, -9.033033306777454641, 21.50000000000000000 ) ) ;
#19063=DIRECTION ( 'NONE',  ( 0.000000000000000000, 1.000000000000000000, 0.000000000000000000 ) ) ;
#19074=VERTEX_POINT ( 'NONE', #18293 ) ;
#19089=EDGE_CURVE ( 'NONE', #9030, #9450, #11430, .T. ) ;
#19108=ORIENTED_EDGE ( 'NONE', *, *, #14661, .T. ) ;
#19110=EDGE_CURVE ( 'NONE', #2495, #15425, #9851, .T. ) ;
#19123=DIRECTION ( 'NONE',  ( 0.000000000000000000, 0.000000000000000000, 1.000000000000000000 ) ) ;
#19126=ORIENTED_EDGE ( 'NONE', *, *, #16652, .F. ) ;
#19128=EDGE_CURVE ( 'NONE', #3416, #14124, #22292, .T. ) ;
#19133=CARTESIAN_POINT ( 'NONE',  ( -7.856594496258223259, -4.390207617113929039, 21.50000000000000000 ) ) ;
#19141=PLANE ( 'NONE',  #21837 ) ;
#19148=VERTEX_POINT ( 'NONE', #24924 ) ;
#19172=EDGE_CURVE ( 'NONE', #19937, #19074, #3375, .T. ) ;
#19188=EDGE_LOOP ( 'NONE', ( #4717, #12535, #1647 ) ) ;
#19198=CARTESIAN_POINT ( 'NONE',  ( 5.069257791428381843, -7.538175180318440027, 13.22130136205108819 ) ) ;
#19200=CARTESIAN_POINT ( 'NONE',  ( -6.364020599487750118, 6.482337650448473099, -1.500000000000001110 ) ) ;
#19210=DIRECTION ( 'NONE',  ( -0.000000000000000000, -0.000000000000000000, 1.000000000000000000 ) ) ;
#19218=AXIS2_PLACEMENT_3D ( 'NONE', #19664, #7824, #26865 ) ;
#19227=VECTOR ( 'NONE', #29578, 1000.000000000000000 ) ;
#19228=ORIENTED_EDGE ( 'NONE', *, *, #8911, .F. ) ;
#19229=ORIENTED_EDGE ( 'NONE', *, *, #15695, .F. ) ;
#19235=ORIENTED_EDGE ( 'NONE', *, *, #10935, .F. ) ;
#19238=CIRCLE ( 'NONE', #11762, 12.18947652193948272 ) ;
#19253=VECTOR ( 'NONE', #29540, 1000.000000000000000 ) ;
#19261=ORIENTED_EDGE ( 'NONE', *, *, #9397, .T. ) ;
#19269=ORIENTED_EDGE ( 'NONE', *, *, #2602, .T. ) ;
#19289=DIRECTION ( 'NONE',  ( 0.000000000000000000, 1.000000000000000000, 0.000000000000000000 ) ) ;
#19298=CARTESIAN_POINT ( 'NONE',  ( -3.196529495465446402, -8.413215745754985875, -3.621320343559650379 ) ) ;
#19301=EDGE_CURVE ( 'NONE', #10553, #25466, #12851, .T. ) ;
#19306=ORIENTED_EDGE ( 'NONE', *, *, #22384, .T. ) ;
#19308=ADVANCED_FACE ( 'NONE', ( #11192 ), #4482, .F. ) ;
#19309=ORIENTED_EDGE ( 'NONE', *, *, #22337, .F. ) ;
#19328=CARTESIAN_POINT ( 'NONE',  ( 0.000000000000000000, -7.422978769709303177E-15, 65.52304386563415051 ) ) ;
#19337=VECTOR ( 'NONE', #15987, 1000.000000000000000 ) ;
#19347=ORIENTED_EDGE ( 'NONE', *, *, #30510, .F. ) ;
#19348=DIRECTION ( 'NONE',  ( 0.000000000000000000, 1.000000000000000000, 0.000000000000000000 ) ) ;
#19352=ORIENTED_EDGE ( 'NONE', *, *, #25991, .F. ) ;
#19354=ORIENTED_EDGE ( 'NONE', *, *, #13347, .T. ) ;
#19366=CARTESIAN_POINT ( 'NONE',  ( -0.8750451464063155882, -9.041888939645136958, 21.50000000000000000 ) ) ;
#19378=CARTESIAN_POINT ( 'NONE',  ( -2.516121109503243858, -8.728722367416578365, 21.50000000000000000 ) ) ;
#19388=ORIENTED_EDGE ( 'NONE', *, *, #11258, .F. ) ;
#19395=AXIS2_PLACEMENT_3D ( 'NONE', #28944, #19576, #394 ) ;
#19416=CYLINDRICAL_SURFACE ( 'NONE', #28047, 0.7500000000000006661 ) ;
#19425=LINE ( 'NONE', #5234, #12440 ) ;
#19431=DIRECTION ( 'NONE',  ( -0.000000000000000000, -0.000000000000000000, 1.000000000000000000 ) ) ;
#19438=ORIENTED_EDGE ( 'NONE', *, *, #16781, .T. ) ;
#19445=DIRECTION ( 'NONE',  ( -0.000000000000000000, -0.000000000000000000, 1.000000000000000000 ) ) ;
#19448=ORIENTED_EDGE ( 'NONE', *, *, #26344, .T. ) ;
#19450=CARTESIAN_POINT ( 'NONE',  ( 0.000000000000000000, -2.435693370351110282E-15, 21.50000000000000355 ) ) ;
#19469=ORIENTED_EDGE ( 'NONE', *, *, #5920, .T. ) ;
#19480=DIRECTION ( 'NONE',  ( 0.000000000000000000, -1.132880637372608986E-16, 1.000000000000000000 ) ) ;
#19482=VERTEX_POINT ( 'NONE', #7905 ) ;
#19492=DIRECTION ( 'NONE',  ( 0.000000000000000000, 0.000000000000000000, 1.000000000000000000 ) ) ;
#19500=DIRECTION ( 'NONE',  ( 0.000000000000000000, 0.000000000000000000, 1.000000000000000000 ) ) ;
#19503=ORIENTED_EDGE ( 'NONE', *, *, #26310, .T. ) ;
#19509=CIRCLE ( 'NONE', #13539, 9.084132297865673777 ) ;
#19510=CARTESIAN_POINT ( 'NONE',  ( 0.000000000000000000, -2.435693370351110282E-15, 21.50000000000000355 ) ) ;
#19522=AXIS2_PLACEMENT_3D ( 'NONE', #21396, #36, #6457 ) ;
#19537=DIRECTION ( 'NONE',  ( 0.000000000000000000, -1.132880637372608986E-16, 1.000000000000000000 ) ) ;
#19546=ORIENTED_EDGE ( 'NONE', *, *, #16120, .F. ) ;
#19576=DIRECTION ( 'NONE',  ( 0.000000000000000000, 0.000000000000000000, 1.000000000000000000 ) ) ;
#19578=ORIENTED_EDGE ( 'NONE', *, *, #16087, .F. ) ;
#19590=CARTESIAN_POINT ( 'NONE',  ( -8.090471615930056259, 1.687027447297517080, -1.500000000000001776 ) ) ;
#19591=CYLINDRICAL_SURFACE ( 'NONE', #9883, 0.7500000000000011102 ) ;
#19596=DIRECTION ( 'NONE',  ( 0.000000000000000000, 0.000000000000000000, 1.000000000000000000 ) ) ;
#19625=DIRECTION ( 'NONE',  ( -0.000000000000000000, 1.132880637372608986E-16, -1.000000000000000000 ) ) ;
#19631=DIRECTION ( 'NONE',  ( 0.000000000000000000, 0.000000000000000000, 1.000000000000000000 ) ) ;
#19637=CIRCLE ( 'NONE', #24630, 9.084132297865673777 ) ;
#19654=CARTESIAN_POINT ( 'NONE',  ( 0.6210184355499436260, -9.062880100047301823, 21.50000000000000000 ) ) ;
#19657=AXIS2_PLACEMENT_3D ( 'NONE', #24913, #22871, #8391 ) ;
#19662=VERTEX_POINT ( 'NONE', #3682 ) ;
#19664=CARTESIAN_POINT ( 'NONE',  ( 0.000000000000000000, -2.435693370351110282E-15, 21.50000000000000355 ) ) ;
#19674=CARTESIAN_POINT ( 'NONE',  ( -1.687027447297492211, -8.840471615930066918, -3.621320343559650379 ) ) ;
#19687=VERTEX_POINT ( 'NONE', #18181 ) ;
#19689=VERTEX_POINT ( 'NONE', #11313 ) ;
#19691=VERTEX_POINT ( 'NONE', #6318 ) ;
#19693=EDGE_CURVE ( 'NONE', #5849, #9666, #8972, .T. ) ;
#19737=FACE_OUTER_BOUND ( 'NONE', #20504, .T. ) ;
#19738=ORIENTED_EDGE ( 'NONE', *, *, #15129, .F. ) ;
#19743=CARTESIAN_POINT ( 'NONE',  ( -1.687027447297492211, -8.840471615930066918, -1.500000000000002665 ) ) ;
#19752=EDGE_LOOP ( 'NONE', ( #7059, #22796, #17485, #2653 ) ) ;
#19753=AXIS2_PLACEMENT_3D ( 'NONE', #20763, #11267, #13477 ) ;
#19780=LINE ( 'NONE', #7953, #2407 ) ;
#19786=DIRECTION ( 'NONE',  ( 0.000000000000000000, 1.000000000000000000, 0.000000000000000000 ) ) ;
#19796=CARTESIAN_POINT ( 'NONE',  ( -6.974883619896829146, -5.687793815610328707, 21.50000000000000000 ) ) ;
#19809=ORIENTED_EDGE ( 'NONE', *, *, #29614, .T. ) ;
#19812=AXIS2_PLACEMENT_3D ( 'NONE', #6659, #11360, #9014 ) ;
#19827=DIRECTION ( 'NONE',  ( -0.000000000000000000, 1.132880637372608986E-16, -1.000000000000000000 ) ) ;
#19851=EDGE_CURVE ( 'NONE', #17197, #1661, #25655, .T. ) ;
#19863=DIRECTION ( 'NONE',  ( -0.000000000000000000, 1.132880637372608986E-16, -1.000000000000000000 ) ) ;
#19864=CIRCLE ( 'NONE', #14380, 0.7499999999999997780 ) ;
#19871=LINE ( 'NONE', #7717, #4659 ) ;
#19876=DIRECTION ( 'NONE',  ( 0.000000000000000000, 1.000000000000000000, 1.193512090021232842E-16 ) ) ;
#19878=EDGE_CURVE ( 'NONE', #19148, #897, #12353, .T. ) ;
#19894=EDGE_CURVE ( 'NONE', #5002, #13097, #11380, .T. ) ;
#19904=EDGE_CURVE ( 'NONE', #18015, #7211, #7882, .T. ) ;
#19907=CIRCLE ( 'NONE', #17930, 0.7499999999999988898 ) ;
#19915=CARTESIAN_POINT ( 'NONE',  ( 0.000000000000000000, -2.435693370351110282E-15, 21.50000000000000355 ) ) ;
#19919=DIRECTION ( 'NONE',  ( 0.000000000000000000, 1.000000000000000000, 1.132880637372608986E-16 ) ) ;
#19920=ORIENTED_EDGE ( 'NONE', *, *, #4464, .F. ) ;
#19925=ORIENTED_EDGE ( 'NONE', *, *, #27287, .F. ) ;
#19927=EDGE_CURVE ( 'NONE', #16535, #29624, #9362, .T. ) ;
#19937=VERTEX_POINT ( 'NONE', #27193 ) ;
#19950=CARTESIAN_POINT ( 'NONE',  ( -0.7083562926194498788, 9.056472324687614872, -1.500000000000000666 ) ) ;
#19959=PLANE ( 'NONE',  #10872 ) ;
#19961=CARTESIAN_POINT ( 'NONE',  ( 0.000000000000000000, -2.435693370351110282E-15, 21.50000000000000355 ) ) ;
#19963=CARTESIAN_POINT ( 'NONE',  ( -0.6210184355500070197, 9.062880100047294718, 21.50000000000000000 ) ) ;
#19964=EDGE_CURVE ( 'NONE', #16535, #12192, #15324, .T. ) ;
#19990=VERTEX_POINT ( 'NONE', #24381 ) ;
#19994=DIRECTION ( 'NONE',  ( 0.000000000000000000, -1.132880637372608986E-16, 1.000000000000000000 ) ) ;
#19996=DIRECTION ( 'NONE',  ( 0.000000000000000000, 0.000000000000000000, 1.000000000000000000 ) ) ;
#19999=AXIS2_PLACEMENT_3D ( 'NONE', #10551, #17890, #3691 ) ;
#20003=VERTEX_POINT ( 'NONE', #3491 ) ;
#20018=AXIS2_PLACEMENT_3D ( 'NONE', #6012, #3361, #15519 ) ;
#20025=CARTESIAN_POINT ( 'NONE',  ( -8.159193615868369776, 3.993622308618967498, 21.50000000000000000 ) ) ;
#20028=EDGE_CURVE ( 'NONE', #12636, #11838, #8806, .T. ) ;
#20033=EDGE_CURVE ( 'NONE', #29057, #7554, #4807, .T. ) ;
#20040=EDGE_CURVE ( 'NONE', #23603, #26525, #8373, .T. ) ;
#20051=VECTOR ( 'NONE', #20709, 1000.000000000000000 ) ;
#20056=CARTESIAN_POINT ( 'NONE',  ( -0.7083562926194498788, 9.056472324687613096, 13.22130136205108997 ) ) ;
#20059=FACE_OUTER_BOUND ( 'NONE', #8627, .T. ) ;
#20064=CARTESIAN_POINT ( 'NONE',  ( -5.131244434206278626, -6.812559277181949646, 21.50000000000000000 ) ) ;
#20067=EDGE_CURVE ( 'NONE', #20761, #12360, #15841, .T. ) ;
#20082=CARTESIAN_POINT ( 'NONE',  ( 7.392982946727082449, -5.278755796068694828, 21.50000000000000000 ) ) ;
#20096=ADVANCED_FACE ( 'NONE', ( #27818 ), #8772, .F. ) ;
#20151=VERTEX_POINT ( 'NONE', #2363 ) ;
#20153=CARTESIAN_POINT ( 'NONE',  ( 0.000000000000000000, 0.000000000000000000, -87.50000000000000000 ) ) ;
#20156=EDGE_LOOP ( 'NONE', ( #21425, #15556, #30431, #11949 ) ) ;
#20161=AXIS2_PLACEMENT_3D ( 'NONE', #28297, #6921, #2229 ) ;
#20169=VERTEX_POINT ( 'NONE', #5167 ) ;
#20178=AXIS2_PLACEMENT_3D ( 'NONE', #20153, #25302, #22342 ) ;
#20186=CARTESIAN_POINT ( 'NONE',  ( 0.000000000000000000, 10.00000000000000888, 117.5000000000000000 ) ) ;
#20188=EDGE_CURVE ( 'NONE', #23298, #21957, #11305, .T. ) ;
#20190=CARTESIAN_POINT ( 'NONE',  ( -7.730328572437709767, 4.608906612435681005, -1.500000000000001332 ) ) ;
#20197=VECTOR ( 'NONE', #7530, 1000.000000000000000 ) ;
#20206=CARTESIAN_POINT ( 'NONE',  ( 0.000000000000000000, -1.324687536737320328E-14, 29.43090101791767665 ) ) ;
#20207=ORIENTED_EDGE ( 'NONE', *, *, #23274, .F. ) ;
#20211=CIRCLE ( 'NONE', #2807, 0.7500000000000006661 ) ;
#20213=ORIENTED_EDGE ( 'NONE', *, *, #10902, .F. ) ;
#20214=ADVANCED_FACE ( 'NONE', ( #14055 ), #9537, .T. ) ;
#20223=CIRCLE ( 'NONE', #27717, 0.7500000000000006661 ) ;
#20247=CYLINDRICAL_SURFACE ( 'NONE', #24481, 15.00000000000003375 ) ;
#20255=CIRCLE ( 'NONE', #5811, 9.084132297865673777 ) ;
#20261=CARTESIAN_POINT ( 'NONE',  ( 1.112485354161228957E-15, -9.084132297865677330, 27.94260272410217638 ) ) ;
#20268=CARTESIAN_POINT ( 'NONE',  ( -6.812559277181930106, 5.881244434206302607, 21.50000000000000000 ) ) ;
#20270=DIRECTION ( 'NONE',  ( 1.000000000000000000, 0.000000000000000000, 0.000000000000000000 ) ) ;
#20280=CIRCLE ( 'NONE', #6820, 9.084132297865673777 ) ;
#20300=ORIENTED_EDGE ( 'NONE', *, *, #13412, .T. ) ;
#20312=ORIENTED_EDGE ( 'NONE', *, *, #20976, .F. ) ;
#20313=AXIS2_PLACEMENT_3D ( 'NONE', #30749, #11891, #2367 ) ;
#20317=CYLINDRICAL_SURFACE ( 'NONE', #20178, 12.18947652193948272 ) ;
#20320=ORIENTED_EDGE ( 'NONE', *, *, #25764, .F. ) ;
#20335=CARTESIAN_POINT ( 'NONE',  ( 0.000000000000000000, 1.699320956058915452E-16, -1.500000000000001776 ) ) ;
#20358=AXIS2_PLACEMENT_3D ( 'NONE', #24980, #22793, #3471 ) ;
#20360=ORIENTED_EDGE ( 'NONE', *, *, #18398, .T. ) ;
#20379=ORIENTED_EDGE ( 'NONE', *, *, #30529, .F. ) ;
#20386=CARTESIAN_POINT ( 'NONE',  ( 8.268028093133366951, 3.763133143576461670, 13.22130136205108819 ) ) ;
#20401=DIRECTION ( 'NONE',  ( 0.000000000000000000, -1.132880637372608986E-16, 1.000000000000000000 ) ) ;
#20407=DIRECTION ( 'NONE',  ( -9.830099697201897928E-15, 1.000000000000000000, 0.000000000000000000 ) ) ;
#20410=ORIENTED_EDGE ( 'NONE', *, *, #14898, .F. ) ;
#20415=ORIENTED_EDGE ( 'NONE', *, *, #13635, .F. ) ;
#20416=ORIENTED_EDGE ( 'NONE', *, *, #9780, .T. ) ;
#20419=DIRECTION ( 'NONE',  ( 1.000000000000000000, 0.000000000000000000, 0.000000000000000000 ) ) ;
#20445=DIRECTION ( 'NONE',  ( 1.000000000000000000, 0.000000000000000000, 0.000000000000000000 ) ) ;
#20447=DIRECTION ( 'NONE',  ( -0.000000000000000000, 1.132880637372608986E-16, -1.000000000000000000 ) ) ;
#20453=EDGE_LOOP ( 'NONE', ( #21994, #26658, #18516, #2944 ) ) ;
#20470=DIRECTION ( 'NONE',  ( -0.000000000000000000, 1.132880637372608986E-16, -1.000000000000000000 ) ) ;
#20471=CIRCLE ( 'NONE', #13581, 9.084132297865673777 ) ;
#20477=DIRECTION ( 'NONE',  ( 1.000000000000000000, 0.000000000000000000, 0.000000000000000000 ) ) ;
#20485=DIRECTION ( 'NONE',  ( 0.000000000000000000, 1.132880637372608986E-16, -1.000000000000000000 ) ) ;
#20504=EDGE_LOOP ( 'NONE', ( #9176, #18094, #16374 ) ) ;
#20512=CYLINDRICAL_SURFACE ( 'NONE', #30783, 12.50000000000000000 ) ;
#20519=FACE_OUTER_BOUND ( 'NONE', #12673, .T. ) ;
#20521=CARTESIAN_POINT ( 'NONE',  ( -3.763133143576374628, 8.268028093133407808, 21.50000000000000000 ) ) ;
#20522=DIRECTION ( 'NONE',  ( 0.000000000000000000, -1.132880637372608986E-16, 1.000000000000000000 ) ) ;
#20523=VERTEX_POINT ( 'NONE', #1022 ) ;
#20524=EDGE_LOOP ( 'NONE', ( #20688, #7523, #20708 ) ) ;
#20536=LINE ( 'NONE', #26097, #28199 ) ;
#20538=CARTESIAN_POINT ( 'NONE',  ( -8.884323311075783991, -1.438332125858144295, 21.50000000000000000 ) ) ;
#20541=AXIS2_PLACEMENT_3D ( 'NONE', #19961, #5621, #8116 ) ;
#20551=PLANE ( 'NONE',  #26491 ) ;
#20568=ORIENTED_EDGE ( 'NONE', *, *, #23523, .F. ) ;
#20586=EDGE_CURVE ( 'NONE', #25466, #9598, #12303, .T. ) ;
#20601=ADVANCED_FACE ( 'NONE', ( #29560, #5695 ), #15190, .T. ) ;
#20602=AXIS2_PLACEMENT_3D ( 'NONE', #430, #9948, #24285 ) ;
#20604=DIRECTION ( 'NONE',  ( 0.000000000000000000, -1.132880637372608986E-16, 1.000000000000000000 ) ) ;
#20611=CARTESIAN_POINT ( 'NONE',  ( 0.000000000000000000, -2.435693370351110282E-15, 21.50000000000000355 ) ) ;
#20612=EDGE_LOOP ( 'NONE', ( #14147, #27422 ) ) ;
#20616=DIRECTION ( 'NONE',  ( 1.000000000000000000, 0.000000000000000000, 0.000000000000000000 ) ) ;
#20621=EDGE_CURVE ( 'NONE', #16043, #1665, #8762, .T. ) ;
#20632=DIRECTION ( 'NONE',  ( 0.000000000000000000, 0.000000000000000000, 1.000000000000000000 ) ) ;
#20635=DIRECTION ( 'NONE',  ( 0.000000000000000000, 0.000000000000000000, 1.000000000000000000 ) ) ;
#20638=DIRECTION ( 'NONE',  ( 0.000000000000000000, 0.000000000000000000, 1.000000000000000000 ) ) ;
#20650=ORIENTED_EDGE ( 'NONE', *, *, #23486, .T. ) ;
#20653=EDGE_LOOP ( 'NONE', ( #13805, #24347, #18267, #27285 ) ) ;
#20666=AXIS2_PLACEMENT_3D ( 'NONE', #12570, #10065, #5692 ) ;
#20668=DIRECTION ( 'NONE',  ( 0.000000000000000000, 1.000000000000000000, 1.193512090021232842E-16 ) ) ;
#20673=PLANE ( 'NONE',  #23403 ) ;
#20685=ORIENTED_EDGE ( 'NONE', *, *, #13613, .T. ) ;
#20688=ORIENTED_EDGE ( 'NONE', *, *, #28055, .F. ) ;
#20692=CYLINDRICAL_SURFACE ( 'NONE', #17321, 0.7499999999999988898 ) ;
#20701=ORIENTED_EDGE ( 'NONE', *, *, #17756, .T. ) ;
#20708=ORIENTED_EDGE ( 'NONE', *, *, #6966, .F. ) ;
#20709=DIRECTION ( 'NONE',  ( -0.000000000000000000, 1.132880637372608986E-16, -1.000000000000000000 ) ) ;
#20718=VERTEX_POINT ( 'NONE', #28557 ) ;
#20726=VECTOR ( 'NONE', #15079, 1000.000000000000000 ) ;
#20749=ORIENTED_EDGE ( 'NONE', *, *, #13398, .T. ) ;
#20758=ADVANCED_FACE ( 'NONE', ( #23408 ), #1742, .F. ) ;
#20761=VERTEX_POINT ( 'NONE', #28408 ) ;
#20763=CARTESIAN_POINT ( 'NONE',  ( -6.974883619896829146, -5.687793815610328707, -3.621320343559650379 ) ) ;
#20765=CARTESIAN_POINT ( 'NONE',  ( 0.000000000000000000, -2.435693370351110282E-15, 21.50000000000000355 ) ) ;
#20775=DIRECTION ( 'NONE',  ( -0.000000000000000000, 1.132880637372608986E-16, -1.000000000000000000 ) ) ;
#20782=EDGE_CURVE ( 'NONE', #27491, #18015, #21057, .T. ) ;
#20788=EDGE_CURVE ( 'NONE', #5755, #9461, #17307, .T. ) ;
#20798=AXIS2_PLACEMENT_3D ( 'NONE', #3560, #13083, #22572 ) ;
#20807=VECTOR ( 'NONE', #4248, 1000.000000000000000 ) ;
#20808=CARTESIAN_POINT ( 'NONE',  ( 0.7083562926195156040, -9.056472324687613096, 13.22130136205108641 ) ) ;
#20810=LINE ( 'NONE', #18182, #23781 ) ;
#20812=VERTEX_POINT ( 'NONE', #12027 ) ;
#20815=CARTESIAN_POINT ( 'NONE',  ( 8.817355867515813017, 2.185336383880231548, 13.22130136205108819 ) ) ;
#20821=DIRECTION ( 'NONE',  ( 0.000000000000000000, 1.000000000000000000, 0.000000000000000000 ) ) ;
#20826=LINE ( 'NONE', #8991, #17070 ) ;
#20833=ADVANCED_FACE ( 'NONE', ( #7189 ), #12498, .F. ) ;
#20841=EDGE_CURVE ( 'NONE', #9598, #10553, #28264, .T. ) ;
#20847=ORIENTED_EDGE ( 'NONE', *, *, #24263, .T. ) ;
#20856=AXIS2_PLACEMENT_3D ( 'NONE', #2036, #21050, #13462 ) ;
#20865=VECTOR ( 'NONE', #10413, 1000.000000000000000 ) ;
#20873=DIRECTION ( 'NONE',  ( 0.000000000000000000, -1.132880637372608986E-16, 1.000000000000000000 ) ) ;
#20877=AXIS2_PLACEMENT_3D ( 'NONE', #24734, #30040, #19919 ) ;
#20879=ORIENTED_EDGE ( 'NONE', *, *, #12798, .T. ) ;
#20899=EDGE_CURVE ( 'NONE', #18134, #4256, #22290, .T. ) ;
#20907=ORIENTED_EDGE ( 'NONE', *, *, #11263, .F. ) ;
#20925=ORIENTED_EDGE ( 'NONE', *, *, #18731, .T. ) ;
#20976=EDGE_CURVE ( 'NONE', #21169, #4121, #27266, .T. ) ;
#21004=ORIENTED_EDGE ( 'NONE', *, *, #15663, .T. ) ;
#21008=FACE_OUTER_BOUND ( 'NONE', #15073, .T. ) ;
#21014=DIRECTION ( 'NONE',  ( 1.000000000000000000, 0.000000000000000000, 0.000000000000000000 ) ) ;
#21022=EDGE_CURVE ( 'NONE', #7139, #20003, #9185, .T. ) ;
#21027=EDGE_CURVE ( 'NONE', #17876, #1692, #23771, .T. ) ;
#21028=VERTEX_POINT ( 'NONE', #6687 ) ;
#21033=EDGE_CURVE ( 'NONE', #29154, #28301, #356, .T. ) ;
#21047=FACE_OUTER_BOUND ( 'NONE', #17731, .T. ) ;
#21050=DIRECTION ( 'NONE',  ( -0.000000000000000000, -0.000000000000000000, 1.000000000000000000 ) ) ;
#21057=LINE ( 'NONE', #21204, #15290 ) ;
#21064=ORIENTED_EDGE ( 'NONE', *, *, #4227, .F. ) ;
#21066=AXIS2_PLACEMENT_3D ( 'NONE', #51, #11748, #2390 ) ;
#21067=DIRECTION ( 'NONE',  ( 0.000000000000000000, 0.000000000000000000, 1.000000000000000000 ) ) ;
#21072=ORIENTED_EDGE ( 'NONE', *, *, #29471, .F. ) ;
#21074=AXIS2_PLACEMENT_3D ( 'NONE', #17528, #525, #5214 ) ;
#21078=FACE_OUTER_BOUND ( 'NONE', #2061, .T. ) ;
#21079=AXIS2_PLACEMENT_3D ( 'NONE', #8262, #15110, #26990 ) ;
#21100=VECTOR ( 'NONE', #11178, 1000.000000000000000 ) ;
#21140=AXIS2_PLACEMENT_3D ( 'NONE', #23475, #2437, #23333 ) ;
#21149=FACE_OUTER_BOUND ( 'NONE', #4809, .T. ) ;
#21166=ORIENTED_EDGE ( 'NONE', *, *, #21494, .F. ) ;
#21169=VERTEX_POINT ( 'NONE', #12467 ) ;
#21179=DIRECTION ( 'NONE',  ( 0.000000000000000000, 1.000000000000000000, 1.193512090021232842E-16 ) ) ;
#21189=CARTESIAN_POINT ( 'NONE',  ( -5.881244434206279514, -6.812559277181949646, 21.50000000000000000 ) ) ;
#21196=VERTEX_POINT ( 'NONE', #25071 ) ;
#21203=VECTOR ( 'NONE', #9508, 1000.000000000000000 ) ;
#21204=CARTESIAN_POINT ( 'NONE',  ( -5.131244434206278626, -6.812559277181949646, -3.621320343559650379 ) ) ;
#21209=DIRECTION ( 'NONE',  ( 1.000000000000000000, 0.000000000000000000, 0.000000000000000000 ) ) ;
#21210=ORIENTED_EDGE ( 'NONE', *, *, #22538, .T. ) ;
#21218=CIRCLE ( 'NONE', #4803, 0.7500000000000006661 ) ;
#21221=CARTESIAN_POINT ( 'NONE',  ( 6.301234758012599357, -6.543385983536367689, -1.500000000000002442 ) ) ;
#21222=ORIENTED_EDGE ( 'NONE', *, *, #13635, .T. ) ;
#21227=FACE_OUTER_BOUND ( 'NONE', #18205, .T. ) ;
#21234=CARTESIAN_POINT ( 'NONE',  ( -2.516121109503243414, -8.728722367416576589, -1.500000000000002887 ) ) ;
#21242=AXIS2_PLACEMENT_3D ( 'NONE', #11768, #21268, #11168 ) ;
#21248=CARTESIAN_POINT ( 'NONE',  ( 6.812559277181973627, -5.881244434206257310, -3.621320343559650379 ) ) ;
#21268=DIRECTION ( 'NONE',  ( 0.000000000000000000, 0.000000000000000000, 1.000000000000000000 ) ) ;
#21269=DIRECTION ( 'NONE',  ( -0.000000000000000000, 1.132880637372608986E-16, -1.000000000000000000 ) ) ;
#21280=AXIS2_PLACEMENT_3D ( 'NONE', #7695, #2851, #7540 ) ;
#21301=DIRECTION ( 'NONE',  ( -0.000000000000000000, 1.132880637372608986E-16, -1.000000000000000000 ) ) ;
#21302=CARTESIAN_POINT ( 'NONE',  ( -1.438332125858111432, 8.884323311075791096, 21.50000000000000000 ) ) ;
#21304=ORIENTED_EDGE ( 'NONE', *, *, #21611, .F. ) ;
#21314=ORIENTED_EDGE ( 'NONE', *, *, #620, .F. ) ;
#21318=CARTESIAN_POINT ( 'NONE',  ( -5.278755796068719697, -7.392982946727062021, -1.500000000000002665 ) ) ;
#21321=EDGE_LOOP ( 'NONE', ( #7506, #22864, #19354, #25261 ) ) ;
#21334=ORIENTED_EDGE ( 'NONE', *, *, #17564, .F. ) ;
#21339=VECTOR ( 'NONE', #16649, 1000.000000000000000 ) ;
#21340=CIRCLE ( 'NONE', #26846, 0.7500000000000007772 ) ;
#21341=ORIENTED_EDGE ( 'NONE', *, *, #823, .T. ) ;
#21342=CARTESIAN_POINT ( 'NONE',  ( 0.000000000000000000, 1.699320956058915452E-16, -1.500000000000001776 ) ) ;
#21345=CARTESIAN_POINT ( 'NONE',  ( 0.000000000000000000, 1.699320956058915452E-16, -1.500000000000001776 ) ) ;
#21348=EDGE_CURVE ( 'NONE', #28044, #2431, #5868, .T. ) ;
#21358=ORIENTED_EDGE ( 'NONE', *, *, #9534, .T. ) ;
#21361=EDGE_CURVE ( 'NONE', #1033, #19689, #18378, .T. ) ;
#21372=CIRCLE ( 'NONE', #2461, 9.084132297865673777 ) ;
#21375=CARTESIAN_POINT ( 'NONE',  ( 7.856594496258195726, 4.390207617113981442, 21.50000000000000000 ) ) ;
#21383=DIRECTION ( 'NONE',  ( -0.000000000000000000, 1.132880637372608986E-16, -1.000000000000000000 ) ) ;
#21386=CARTESIAN_POINT ( 'NONE',  ( -4.608906612435655248, -7.730328572437724866, 21.50000000000000000 ) ) ;
#21387=LINE ( 'NONE', #6740, #25321 ) ;
#21388=EDGE_CURVE ( 'NONE', #9030, #2587, #7879, .T. ) ;
#21396=CARTESIAN_POINT ( 'NONE',  ( -7.856594496258223259, -4.390207617113929039, -3.621320343559650379 ) ) ;
#21404=DIRECTION ( 'NONE',  ( -0.000000000000000000, -0.000000000000000000, 1.000000000000000000 ) ) ;
#21425=ORIENTED_EDGE ( 'NONE', *, *, #9795, .F. ) ;
#21438=CARTESIAN_POINT ( 'NONE',  ( -7.106594496258223259, -4.390207617113929039, -3.621320343559650379 ) ) ;
#21445=LINE ( 'NONE', #16766, #24587 ) ;
#21456=DIRECTION ( 'NONE',  ( 0.000000000000000000, 1.000000000000000000, 1.193512090021232842E-16 ) ) ;
#21461=VERTEX_POINT ( 'NONE', #28344 ) ;
#21473=ORIENTED_EDGE ( 'NONE', *, *, #6869, .T. ) ;
#21479=AXIS2_PLACEMENT_3D ( 'NONE', #30039, #27086, #18191 ) ;
#21494=EDGE_CURVE ( 'NONE', #699, #2118, #13389, .T. ) ;
#21516=FACE_OUTER_BOUND ( 'NONE', #12617, .T. ) ;
#21519=ORIENTED_EDGE ( 'NONE', *, *, #13464, .T. ) ;
#21535=DIRECTION ( 'NONE',  ( -0.000000000000000000, 1.132880637372608986E-16, -1.000000000000000000 ) ) ;
#21542=VERTEX_POINT ( 'NONE', #7434 ) ;
#21554=CIRCLE ( 'NONE', #8132, 0.7500000000000006661 ) ;
#21555=ORIENTED_EDGE ( 'NONE', *, *, #16744, .T. ) ;
#21561=EDGE_CURVE ( 'NONE', #1314, #21169, #6389, .T. ) ;
#21568=ORIENTED_EDGE ( 'NONE', *, *, #12580, .T. ) ;
#21586=DIRECTION ( 'NONE',  ( 1.000000000000000000, 0.000000000000000000, 0.000000000000000000 ) ) ;
#21607=AXIS2_PLACEMENT_3D ( 'NONE', #9687, #6889, #4546 ) ;
#21611=EDGE_CURVE ( 'NONE', #5849, #21196, #7365, .T. ) ;
#21614=CARTESIAN_POINT ( 'NONE',  ( 0.000000000000000000, 1.699320956058915452E-16, -1.500000000000001776 ) ) ;
#21615=EDGE_CURVE ( 'NONE', #23454, #28205, #13360, .T. ) ;
#21616=DIRECTION ( 'NONE',  ( 0.000000000000000000, 0.000000000000000000, 1.000000000000000000 ) ) ;
#21618=ORIENTED_EDGE ( 'NONE', *, *, #26310, .F. ) ;
#21672=ORIENTED_EDGE ( 'NONE', *, *, #17580, .T. ) ;
#21688=FACE_OUTER_BOUND ( 'NONE', #6880, .T. ) ;
#21695=ORIENTED_EDGE ( 'NONE', *, *, #29443, .T. ) ;
#21696=DIRECTION ( 'NONE',  ( 1.000000000000000000, 0.000000000000000000, 0.000000000000000000 ) ) ;
#21701=DIRECTION ( 'NONE',  ( 0.000000000000000000, 1.000000000000000000, 0.000000000000000000 ) ) ;
#21714=CARTESIAN_POINT ( 'NONE',  ( 9.062880100047298271, 0.6210184355499750453, -1.500000000000001776 ) ) ;
#21718=ORIENTED_EDGE ( 'NONE', *, *, #1909, .T. ) ;
#21723=DIRECTION ( 'NONE',  ( 0.000000000000000000, 1.000000000000000000, 1.193512090021232842E-16 ) ) ;
#21732=CIRCLE ( 'NONE', #3826, 0.7499999999999997780 ) ;
#21757=EDGE_CURVE ( 'NONE', #15951, #16368, #901, .T. ) ;
#21758=ORIENTED_EDGE ( 'NONE', *, *, #5428, .F. ) ;
#21766=EDGE_LOOP ( 'NONE', ( #2107, #141, #19261, #26420 ) ) ;
#21783=ORIENTED_EDGE ( 'NONE', *, *, #11577, .T. ) ;
#21804=ORIENTED_EDGE ( 'NONE', *, *, #17175, .T. ) ;
#21819=ORIENTED_EDGE ( 'NONE', *, *, #15449, .F. ) ;
#21829=DIRECTION ( 'NONE',  ( 1.000000000000000000, 0.000000000000000000, -0.000000000000000000 ) ) ;
#21837=AXIS2_PLACEMENT_3D ( 'NONE', #3070, #12593, #17104 ) ;
#21841=VERTEX_POINT ( 'NONE', #22990 ) ;
#21846=AXIS2_PLACEMENT_3D ( 'NONE', #17483, #27006, #3278 ) ;
#21847=DIRECTION ( 'NONE',  ( 0.000000000000000000, -1.132880637372608986E-16, 1.000000000000000000 ) ) ;
#21848=ORIENTED_EDGE ( 'NONE', *, *, #6711, .F. ) ;
#21873=ORIENTED_EDGE ( 'NONE', *, *, #24817, .F. ) ;
#21886=DIRECTION ( 'NONE',  ( 0.000000000000000000, -1.132880637372608986E-16, 1.000000000000000000 ) ) ;
#21891=PLANE ( 'NONE',  #30754 ) ;
#21899=DIRECTION ( 'NONE',  ( 0.000000000000000000, 0.000000000000000000, 1.000000000000000000 ) ) ;
#21906=DIRECTION ( 'NONE',  ( 1.000000000000000000, 0.000000000000000000, 0.000000000000000000 ) ) ;
#21928=CARTESIAN_POINT ( 'NONE',  ( 7.856594496258195726, 4.390207617113981442, -1.500000000000001332 ) ) ;
#21931=CIRCLE ( 'NONE', #14965, 0.7500000000000006661 ) ;
#21943=EDGE_CURVE ( 'NONE', #5756, #12636, #11884, .T. ) ;
#21957=VERTEX_POINT ( 'NONE', #9720 ) ;
#21966=DIRECTION ( 'NONE',  ( 1.000000000000000000, 0.000000000000000000, 0.000000000000000000 ) ) ;
#21967=EDGE_CURVE ( 'NONE', #15826, #10427, #5357, .T. ) ;
#21994=ORIENTED_EDGE ( 'NONE', *, *, #20621, .F. ) ;
#22008=CARTESIAN_POINT ( 'NONE',  ( -5.069257791428326776, 7.538175180318475554, -1.500000000000000888 ) ) ;
#22013=DIRECTION ( 'NONE',  ( 0.000000000000000000, 1.000000000000000000, 0.000000000000000000 ) ) ;
#22019=CARTESIAN_POINT ( 'NONE',  ( 3.763133143576435913, -8.268028093133381162, 13.22130136205108641 ) ) ;
#22023=FACE_OUTER_BOUND ( 'NONE', #29061, .T. ) ;
#22034=CARTESIAN_POINT ( 'NONE',  ( -4.608906612435655248, -7.730328572437724866, -1.500000000000002665 ) ) ;
#22036=DIRECTION ( 'NONE',  ( -0.000000000000000000, -0.000000000000000000, 1.000000000000000000 ) ) ;
#22049=VECTOR ( 'NONE', #9097, 1000.000000000000000 ) ;
#22051=DIRECTION ( 'NONE',  ( 1.000000000000000000, 0.000000000000000000, 0.000000000000000000 ) ) ;
#22052=ORIENTED_EDGE ( 'NONE', *, *, #8098, .F. ) ;
#22053=ORIENTED_EDGE ( 'NONE', *, *, #16997, .T. ) ;
#22058=CARTESIAN_POINT ( 'NONE',  ( 1.530808498934191521E-15, -12.50000000000000000, -87.50000000000000000 ) ) ;
#22062=ADVANCED_FACE ( 'NONE', ( #5820 ), #12850, .F. ) ;
#22069=ORIENTED_EDGE ( 'NONE', *, *, #22945, .F. ) ;
#22071=AXIS2_PLACEMENT_3D ( 'NONE', #9969, #7621, #10429 ) ;
#22072=CIRCLE ( 'NONE', #14120, 0.7500000000000006661 ) ;
#22091=CIRCLE ( 'NONE', #21079, 0.7500000000000006661 ) ;
#22111=EDGE_CURVE ( 'NONE', #11519, #6070, #3419, .T. ) ;
#22125=ORIENTED_EDGE ( 'NONE', *, *, #30529, .T. ) ;
#22126=ORIENTED_EDGE ( 'NONE', *, *, #868, .T. ) ;
#22134=DIRECTION ( 'NONE',  ( 0.000000000000000000, -1.132880637372608986E-16, 1.000000000000000000 ) ) ;
#22136=CIRCLE ( 'NONE', #1226, 0.7499999999999997780 ) ;
#22137=EDGE_CURVE ( 'NONE', #2587, #2272, #12696, .T. ) ;
#22152=ADVANCED_FACE ( 'NONE', ( #5158 ), #23442, .F. ) ;
#22171=EDGE_CURVE ( 'NONE', #3179, #12072, #12897, .T. ) ;
#22187=CARTESIAN_POINT ( 'NONE',  ( -8.795879380940579750, -2.270234684139648795, -1.500000000000001998 ) ) ;
#22192=DIRECTION ( 'NONE',  ( -2.312964634635740689E-15, 1.000000000000000000, 0.000000000000000000 ) ) ;
#22223=DIRECTION ( 'NONE',  ( 0.000000000000000000, 0.000000000000000000, 1.000000000000000000 ) ) ;
#22226=ORIENTED_EDGE ( 'NONE', *, *, #20586, .T. ) ;
#22228=AXIS2_PLACEMENT_3D ( 'NONE', #28224, #14175, #26191 ) ;
#22262=ORIENTED_EDGE ( 'NONE', *, *, #23330, .F. ) ;
#22278=CIRCLE ( 'NONE', #8845, 0.7500000000000006661 ) ;
#22289=CARTESIAN_POINT ( 'NONE',  ( 0.000000000000000000, 1.699320956058915452E-16, -1.500000000000001776 ) ) ;
#22290=CIRCLE ( 'NONE', #6835, 9.084132297865673777 ) ;
#22292=CIRCLE ( 'NONE', #10845, 0.7500000000000011102 ) ;
#22294=EDGE_LOOP ( 'NONE', ( #6083, #17994 ) ) ;
#22328=CARTESIAN_POINT ( 'NONE',  ( 0.000000000000000000, -2.435693370351110282E-15, 21.50000000000000355 ) ) ;
#22335=ADVANCED_FACE ( 'NONE', ( #29493 ), #24805, .F. ) ;
#22337=EDGE_CURVE ( 'NONE', #6070, #21841, #13414, .T. ) ;
#22340=DIRECTION ( 'NONE',  ( -0.000000000000000000, 1.132880637372608986E-16, -1.000000000000000000 ) ) ;
#22342=DIRECTION ( 'NONE',  ( 0.000000000000000000, 1.000000000000000000, 0.000000000000000000 ) ) ;
#22353=DIRECTION ( 'NONE',  ( -0.000000000000000000, 1.132880637372608986E-16, -1.000000000000000000 ) ) ;
#22356=DIRECTION ( 'NONE',  ( 0.000000000000000000, 0.000000000000000000, 1.000000000000000000 ) ) ;
#22362=CARTESIAN_POINT ( 'NONE',  ( 0.000000000000000000, 7.500000000000000000, -1.500000000000000444 ) ) ;
#22384=EDGE_CURVE ( 'NONE', #11838, #16268, #27099, .T. ) ;
#22385=VERTEX_POINT ( 'NONE', #22556 ) ;
#22386=DIRECTION ( 'NONE',  ( 1.000000000000000000, 0.000000000000000000, 0.000000000000000000 ) ) ;
#22387=EDGE_CURVE ( 'NONE', #7554, #21542, #18401, .T. ) ;
#22388=AXIS2_PLACEMENT_3D ( 'NONE', #16615, #23777, #7419 ) ;
#22396=ORIENTED_EDGE ( 'NONE', *, *, #21615, .F. ) ;
#22401=FACE_OUTER_BOUND ( 'NONE', #23747, .T. ) ;
#22405=AXIS2_PLACEMENT_3D ( 'NONE', #27453, #26483, #14012 ) ;
#22410=CARTESIAN_POINT ( 'NONE',  ( -6.062559277181930106, 5.881244434206302607, -1.500000000000000888 ) ) ;
#22415=EDGE_CURVE ( 'NONE', #11549, #26020, #22849, .T. ) ;
#22446=DIRECTION ( 'NONE',  ( -0.000000000000000000, -0.000000000000000000, 1.000000000000000000 ) ) ;
#22456=ORIENTED_EDGE ( 'NONE', *, *, #10664, .T. ) ;
#22463=DIRECTION ( 'NONE',  ( 1.000000000000000000, 0.000000000000000000, 0.000000000000000000 ) ) ;
#22471=CARTESIAN_POINT ( 'NONE',  ( -8.090471615930056259, 1.687027447297517080, -3.621320343559650379 ) ) ;
#22478=LINE ( 'NONE', #3157, #24856 ) ;
#22491=DIRECTION ( 'NONE',  ( 0.000000000000000000, 0.000000000000000000, 1.000000000000000000 ) ) ;
#22514=ADVANCED_FACE ( 'NONE', ( #24909 ), #8385, .F. ) ;
#22516=ADVANCED_FACE ( 'NONE', ( #15542 ), #22867, .F. ) ;
#22538=EDGE_CURVE ( 'NONE', #9741, #17647, #24864, .T. ) ;
#22556=CARTESIAN_POINT ( 'NONE',  ( -6.301234758012551396, 6.543385983536412986, -1.500000000000001110 ) ) ;
#22557=EDGE_CURVE ( 'NONE', #24466, #14711, #949, .T. ) ;
#22563=ORIENTED_EDGE ( 'NONE', *, *, #25169, .T. ) ;
#22572=DIRECTION ( 'NONE',  ( 1.000000000000000000, 0.000000000000000000, 0.000000000000000000 ) ) ;
#22580=DIRECTION ( 'NONE',  ( 1.000000000000000000, 0.000000000000000000, -0.000000000000000000 ) ) ;
#22590=CARTESIAN_POINT ( 'NONE',  ( -8.303920738747237351, -3.683253992019803746, -1.500000000000002220 ) ) ;
#22600=ORIENTED_EDGE ( 'NONE', *, *, #10325, .F. ) ;
#22607=VECTOR ( 'NONE', #11592, 1000.000000000000000 ) ;
#22619=FACE_OUTER_BOUND ( 'NONE', #13731, .T. ) ;
#22635=ORIENTED_EDGE ( 'NONE', *, *, #26339, .F. ) ;
#22636=LINE ( 'NONE', #27344, #28938 ) ;
#22639=ORIENTED_EDGE ( 'NONE', *, *, #23113, .T. ) ;
#22657=LINE ( 'NONE', #1306, #19253 ) ;
#22668=DIRECTION ( 'NONE',  ( 1.000000000000000000, 0.000000000000000000, 0.000000000000000000 ) ) ;
#22669=ORIENTED_EDGE ( 'NONE', *, *, #18370, .T. ) ;
#22673=ORIENTED_EDGE ( 'NONE', *, *, #23669, .T. ) ;
#22685=EDGE_CURVE ( 'NONE', #23519, #23603, #13974, .T. ) ;
#22689=AXIS2_PLACEMENT_3D ( 'NONE', #29486, #10758, #24949 ) ;
#22704=DIRECTION ( 'NONE',  ( 0.000000000000000000, 0.000000000000000000, 1.000000000000000000 ) ) ;
#22706=DIRECTION ( 'NONE',  ( 0.000000000000000000, -1.132880637372608986E-16, 1.000000000000000000 ) ) ;
#22708=PLANE ( 'NONE',  #7706 ) ;
#22717=LINE ( 'NONE', #13387, #12998 ) ;
#22721=CARTESIAN_POINT ( 'NONE',  ( 0.000000000000000000, -2.435693370351110282E-15, 21.50000000000000355 ) ) ;
#22735=CARTESIAN_POINT ( 'NONE',  ( 0.8750451464062526385, 9.041888939645140510, -1.500000000000000666 ) ) ;
#22742=ORIENTED_EDGE ( 'NONE', *, *, #7655, .T. ) ;
#22762=VECTOR ( 'NONE', #12974, 1000.000000000000000 ) ;
#22763=EDGE_CURVE ( 'NONE', #4121, #21028, #8420, .T. ) ;
#22764=CIRCLE ( 'NONE', #12335, 9.084132297865673777 ) ;
#22772=ORIENTED_EDGE ( 'NONE', *, *, #19904, .F. ) ;
#22787=CARTESIAN_POINT ( 'NONE',  ( -7.392982946727046034, 5.278755796068742789, -1.500000000000001110 ) ) ;
#22792=DIRECTION ( 'NONE',  ( -0.000000000000000000, 1.132880637372608986E-16, -1.000000000000000000 ) ) ;
#22793=DIRECTION ( 'NONE',  ( -0.000000000000000000, -0.000000000000000000, 1.000000000000000000 ) ) ;
#22796=ORIENTED_EDGE ( 'NONE', *, *, #9795, .T. ) ;
#22806=AXIS2_PLACEMENT_3D ( 'NONE', #21614, #9761, #10073 ) ;
#22808=DIRECTION ( 'NONE',  ( 0.000000000000000000, 0.000000000000000000, 1.000000000000000000 ) ) ;
#22810=CARTESIAN_POINT ( 'NONE',  ( 4.608906612435600181, 7.730328572437758616, 21.50000000000000000 ) ) ;
#22812=ADVANCED_FACE ( 'NONE', ( #7731 ), #17230, .F. ) ;
#22823=CARTESIAN_POINT ( 'NONE',  ( 0.000000000000000000, 12.50000000000000000, -87.50000000000000000 ) ) ;
#22829=VERTEX_POINT ( 'NONE', #26755 ) ;
#22830=DIRECTION ( 'NONE',  ( -0.000000000000000000, -0.000000000000000000, 1.000000000000000000 ) ) ;
#22835=ORIENTED_EDGE ( 'NONE', *, *, #23486, .F. ) ;
#22841=CIRCLE ( 'NONE', #26842, 0.7500000000000006661 ) ;
#22842=AXIS2_PLACEMENT_3D ( 'NONE', #9777, #564, #10084 ) ;
#22844=AXIS2_PLACEMENT_3D ( 'NONE', #4154, #16010, #1056 ) ;
#22849=CIRCLE ( 'NONE', #8930, 9.084132297865673777 ) ;
#22864=ORIENTED_EDGE ( 'NONE', *, *, #22137, .T. ) ;
#22865=FACE_OUTER_BOUND ( 'NONE', #14959, .T. ) ;
#22867=PLANE ( 'NONE',  #14391 ) ;
#22871=DIRECTION ( 'NONE',  ( -0.000000000000000000, -0.000000000000000000, 1.000000000000000000 ) ) ;
#22874=PRODUCT_DEFINITION ( 'UNKNOWN', '', #17365, #22920 ) ;
#22878=CARTESIAN_POINT ( 'NONE',  ( 0.000000000000000000, -3.165563358393047634E-15, 27.94260272410217638 ) ) ;
#22880=CARTESIAN_POINT ( 'NONE',  ( 0.000000000000000000, 7.500000000000007994, -87.50000000000000000 ) ) ;
#22905=DIRECTION ( 'NONE',  ( 0.000000000000000000, 1.000000000000000000, 1.193512090021232842E-16 ) ) ;
#22913=CIRCLE ( 'NONE', #9989, 0.7500000000000006661 ) ;
#22914=EDGE_CURVE ( 'NONE', #19687, #27309, #8478, .T. ) ;
#22917=CARTESIAN_POINT ( 'NONE',  ( 0.000000000000000000, -2.435693370351110282E-15, 21.50000000000000355 ) ) ;
#22920=PRODUCT_DEFINITION_CONTEXT ( 'detailed design', #8205, 'design' ) ;
#22921=ORIENTED_EDGE ( 'NONE', *, *, #17393, .T. ) ;
#22922=ORIENTED_EDGE ( 'NONE', *, *, #23253, .F. ) ;
#22930=ORIENTED_EDGE ( 'NONE', *, *, #17668, .T. ) ;
#22937=CARTESIAN_POINT ( 'NONE',  ( 1.530808498934192310E-15, -12.50000000000000888, -16.50000000000000000 ) ) ;
#22944=CARTESIAN_POINT ( 'NONE',  ( 0.000000000000000000, -2.435693370351110282E-15, 21.50000000000000355 ) ) ;
#22945=EDGE_CURVE ( 'NONE', #2495, #30824, #8755, .T. ) ;
#22953=ORIENTED_EDGE ( 'NONE', *, *, #9534, .F. ) ;
#22956=CARTESIAN_POINT ( 'NONE',  ( 0.000000000000000000, -2.435693370351110282E-15, 21.50000000000000355 ) ) ;
#22959=FACE_OUTER_BOUND ( 'NONE', #17949, .T. ) ;
#22966=ORIENTED_EDGE ( 'NONE', *, *, #13989, .T. ) ;
#22967=CARTESIAN_POINT ( 'NONE',  ( 9.062880100047298271, 0.6210184355499750453, 13.22130136205108819 ) ) ;
#22990=CARTESIAN_POINT ( 'NONE',  ( -5.349779314757642901, -7.341751895053217680, -1.500000000000002665 ) ) ;
#23013=( NAMED_UNIT ( * ) SI_UNIT ( $, .STERADIAN. ) SOLID_ANGLE_UNIT ( ) );
#23023=DIRECTION ( 'NONE',  ( 0.000000000000000000, -1.132880637372608986E-16, 1.000000000000000000 ) ) ;
#23024=AXIS2_PLACEMENT_3D ( 'NONE', #13028, #25334, #1166 ) ;
#23034=CARTESIAN_POINT ( 'NONE',  ( 0.000000000000000000, 0.000000000000000000, -87.50000000000000000 ) ) ;
#23050=DIRECTION ( 'NONE',  ( -0.000000000000000000, 1.132880637372608986E-16, -1.000000000000000000 ) ) ;
#23051=PLANE ( 'NONE',  #8968 ) ;
#23053=CARTESIAN_POINT ( 'NONE',  ( -8.249114229549590505, 0.1262659238205133538, -1.500000000000001776 ) ) ;
#23054=FACE_OUTER_BOUND ( 'NONE', #28106, .T. ) ;
#23099=ADVANCED_FACE ( 'NONE', ( #25901 ), #30724, .F. ) ;
#23108=FACE_OUTER_BOUND ( 'NONE', #23366, .T. ) ;
#23113=EDGE_CURVE ( 'NONE', #6919, #19482, #7026, .T. ) ;
#23115=EDGE_CURVE ( 'NONE', #11459, #25155, #28871, .T. ) ;
#23117=CARTESIAN_POINT ( 'NONE',  ( -7.488956955540436056, -5.141690706682852330, 13.22130136205108819 ) ) ;
#23133=ORIENTED_EDGE ( 'NONE', *, *, #22111, .F. ) ;
#23134=DIRECTION ( 'NONE',  ( 1.000000000000000000, 0.000000000000000000, 0.000000000000000000 ) ) ;
#23140=ORIENTED_EDGE ( 'NONE', *, *, #1623, .F. ) ;
#23154=CIRCLE ( 'NONE', #1773, 0.7500000000000006661 ) ;
#23157=DIRECTION ( 'NONE',  ( 0.000000000000000000, 1.000000000000000000, 0.000000000000000000 ) ) ;
#23159=FACE_OUTER_BOUND ( 'NONE', #15934, .T. ) ;
#23160=ORIENTED_EDGE ( 'NONE', *, *, #20899, .F. ) ;
#23161=CARTESIAN_POINT ( 'NONE',  ( 0.000000000000000000, -2.435693370351110282E-15, 21.50000000000000355 ) ) ;
#23164=ORIENTED_EDGE ( 'NONE', *, *, #10090, .T. ) ;
#23172=ORIENTED_EDGE ( 'NONE', *, *, #7568, .T. ) ;
#23174=CIRCLE ( 'NONE', #24695, 0.7500000000000002220 ) ;
#23181=DIRECTION ( 'NONE',  ( 1.000000000000000000, 0.000000000000000000, 0.000000000000000000 ) ) ;
#23183=CYLINDRICAL_SURFACE ( 'NONE', #12116, 0.7500000000000002220 ) ;
#23185=AXIS2_PLACEMENT_3D ( 'NONE', #6629, #30183, #25660 ) ;
#23205=LINE ( 'NONE', #8729, #2025 ) ;
#23208=AXIS2_PLACEMENT_3D ( 'NONE', #651, #9551, #9863 ) ;
#23226=VECTOR ( 'NONE', #26269, 1000.000000000000000 ) ;
#23229=SHAPE_REPRESENTATION ( 'Slotted Rotor Drive Shaft', ( #7396 ), #11893 ) ;
#23237=CIRCLE ( 'NONE', #26231, 0.7499999999999997780 ) ;
#23240=ORIENTED_EDGE ( 'NONE', *, *, #9962, .F. ) ;
#23243=CARTESIAN_POINT ( 'NONE',  ( -6.974883619896829146, -5.687793815610328707, -1.500000000000002220 ) ) ;
#23245=ORIENTED_EDGE ( 'NONE', *, *, #12865, .F. ) ;
#23253=EDGE_CURVE ( 'NONE', #12636, #34, #8118, .T. ) ;
#23263=CIRCLE ( 'NONE', #6338, 0.7499999999999997780 ) ;
#23265=CARTESIAN_POINT ( 'NONE',  ( 0.000000000000000000, -1.324687536737320328E-14, 29.43090101791767665 ) ) ;
#23274=EDGE_CURVE ( 'NONE', #16043, #22829, #21372, .T. ) ;
#23277=CIRCLE ( 'NONE', #9841, 0.7500000000000006661 ) ;
#23282=CARTESIAN_POINT ( 'NONE',  ( -9.033033306777449312, 0.9621688436940325495, -1.500000000000001554 ) ) ;
#23285=LINE ( 'NONE', #1928, #630 ) ;
#23286=ORIENTED_EDGE ( 'NONE', *, *, #3506, .T. ) ;
#23288=AXIS2_PLACEMENT_3D ( 'NONE', #3401, #2124, #11352 ) ;
#23291=AXIS2_PLACEMENT_3D ( 'NONE', #21302, #23344, #25689 ) ;
#23297=CARTESIAN_POINT ( 'NONE',  ( -8.413215745754975217, 3.196529495465474380, 21.50000000000000000 ) ) ;
#23298=VERTEX_POINT ( 'NONE', #27761 ) ;
#23301=EDGE_CURVE ( 'NONE', #16368, #1375, #3903, .T. ) ;
#23302=DIRECTION ( 'NONE',  ( -2.312964634635740689E-15, 1.000000000000000000, 0.000000000000000000 ) ) ;
#23312=ADVANCED_FACE ( 'NONE', ( #4044 ), #23051, .F. ) ;
#23316=DIRECTION ( 'NONE',  ( -0.000000000000000000, 1.132880637372608986E-16, -1.000000000000000000 ) ) ;
#23330=EDGE_CURVE ( 'NONE', #4711, #18115, #8475, .T. ) ;
#23332=AXIS2_PLACEMENT_3D ( 'NONE', #6668, #11367, #14142 ) ;
#23333=DIRECTION ( 'NONE',  ( 0.000000000000000000, 1.000000000000000000, 1.193512090021232842E-16 ) ) ;
#23344=DIRECTION ( 'NONE',  ( 0.000000000000000000, 0.000000000000000000, 1.000000000000000000 ) ) ;
#23346=DIRECTION ( 'NONE',  ( 1.000000000000000000, 0.000000000000000000, 0.000000000000000000 ) ) ;
#23357=ORIENTED_EDGE ( 'NONE', *, *, #25955, .T. ) ;
#23362=VERTEX_POINT ( 'NONE', #6993 ) ;
#23365=CARTESIAN_POINT ( 'NONE',  ( -3.196529495465446402, -8.413215745754985875, -1.500000000000002665 ) ) ;
#23366=EDGE_LOOP ( 'NONE', ( #3150, #14497, #14411, #3319 ) ) ;
#23371=CARTESIAN_POINT ( 'NONE',  ( -8.197313248159920462, 3.914781618004780306, -1.500000000000001332 ) ) ;
#23372=DIRECTION ( 'NONE',  ( 0.000000000000000000, -1.132880637372608986E-16, 1.000000000000000000 ) ) ;
#23373=ORIENTED_EDGE ( 'NONE', *, *, #16587, .T. ) ;
#23374=DIRECTION ( 'NONE',  ( 1.000000000000000000, 0.000000000000000000, 0.000000000000000000 ) ) ;
#23383=AXIS2_PLACEMENT_3D ( 'NONE', #26062, #2352, #11883 ) ;
#23384=DIRECTION ( 'NONE',  ( 0.000000000000000000, 1.000000000000000000, 1.193512090021232842E-16 ) ) ;
#23387=ORIENTED_EDGE ( 'NONE', *, *, #17557, .T. ) ;
#23390=CARTESIAN_POINT ( 'NONE',  ( -7.730328572437709767, 4.608906612435681005, -3.621320343559650379 ) ) ;
#23398=AXIS2_PLACEMENT_3D ( 'NONE', #24202, #16898, #26414 ) ;
#23403=AXIS2_PLACEMENT_3D ( 'NONE', #29906, #6186, #8222 ) ;
#23405=DIRECTION ( 'NONE',  ( 0.000000000000000000, -1.132880637372608986E-16, 1.000000000000000000 ) ) ;
#23408=FACE_OUTER_BOUND ( 'NONE', #13376, .T. ) ;
#23416=DIRECTION ( 'NONE',  ( 0.000000000000000000, 1.000000000000000000, 0.000000000000000000 ) ) ;
#23422=CARTESIAN_POINT ( 'NONE',  ( 0.000000000000000000, -2.435693370351110282E-15, 21.50000000000000355 ) ) ;
#23427=LINE ( 'NONE', #30456, #22049 ) ;
#23431=LINE ( 'NONE', #27979, #22607 ) ;
#23442=PLANE ( 'NONE',  #26326 ) ;
#23454=VERTEX_POINT ( 'NONE', #18777 ) ;
#23455=DIRECTION ( 'NONE',  ( 0.000000000000000000, -1.132880637372608986E-16, 1.000000000000000000 ) ) ;
#23459=DIRECTION ( 'NONE',  ( -0.000000000000000000, 1.132880637372608986E-16, -1.000000000000000000 ) ) ;
#23461=DIRECTION ( 'NONE',  ( 0.000000000000000000, 1.132880637372608986E-16, -1.000000000000000000 ) ) ;
#23475=CARTESIAN_POINT ( 'NONE',  ( 0.000000000000000000, 1.699320956058915452E-16, -1.500000000000001776 ) ) ;
#23478=ORIENTED_EDGE ( 'NONE', *, *, #17182, .T. ) ;
#23486=EDGE_CURVE ( 'NONE', #9666, #9137, #29882, .T. ) ;
#23490=CARTESIAN_POINT ( 'NONE',  ( 8.499586724479435418, 2.959227181723830036, -3.621320343559650379 ) ) ;
#23494=DIRECTION ( 'NONE',  ( 1.000000000000000000, 0.000000000000000000, 0.000000000000000000 ) ) ;
#23503=AXIS2_PLACEMENT_3D ( 'NONE', #29021, #21847, #16866 ) ;
#23506=EDGE_CURVE ( 'NONE', #5775, #9872, #1493, .T. ) ;
#23509=DIRECTION ( 'NONE',  ( 0.000000000000000000, 1.000000000000000000, 0.000000000000000000 ) ) ;
#23513=ORIENTED_EDGE ( 'NONE', *, *, #22557, .T. ) ;
#23514=AXIS2_PLACEMENT_3D ( 'NONE', #6183, #1808, #15377 ) ;
#23519=VERTEX_POINT ( 'NONE', #28298 ) ;
#23522=ORIENTED_EDGE ( 'NONE', *, *, #7473, .F. ) ;
#23523=EDGE_CURVE ( 'NONE', #23828, #29162, #18917, .T. ) ;
#23541=LINE ( 'NONE', #23689, #26817 ) ;
#23559=DIRECTION ( 'NONE',  ( -0.000000000000000000, -0.000000000000000000, 1.000000000000000000 ) ) ;
#23564=DIRECTION ( 'NONE',  ( -0.000000000000000000, 1.132880637372608986E-16, -1.000000000000000000 ) ) ;
#23587=DIRECTION ( 'NONE',  ( 1.000000000000000000, 0.000000000000000000, 0.000000000000000000 ) ) ;
#23603=VERTEX_POINT ( 'NONE', #13652 ) ;
#23614=CARTESIAN_POINT ( 'NONE',  ( -8.413215745754975217, 3.196529495465474380, -3.621320343559650379 ) ) ;
#23619=ORIENTED_EDGE ( 'NONE', *, *, #28250, .F. ) ;
#23632=FACE_OUTER_BOUND ( 'NONE', #25368, .T. ) ;
#23637=DIRECTION ( 'NONE',  ( 1.000000000000000000, 0.000000000000000000, 0.000000000000000000 ) ) ;
#23656=CARTESIAN_POINT ( 'NONE',  ( 2.270234684139677217, -8.795879380940572645, -1.500000000000002887 ) ) ;
#23657=CIRCLE ( 'NONE', #12212, 0.7499999999999997780 ) ;
#23669=EDGE_CURVE ( 'NONE', #7211, #15632, #28379, .T. ) ;
#23689=CARTESIAN_POINT ( 'NONE',  ( -9.041888939645131629, 0.8750451464063457863, 13.22130136205108819 ) ) ;
#23698=DIRECTION ( 'NONE',  ( -2.312964634635740689E-15, 1.000000000000000000, 0.000000000000000000 ) ) ;
#23703=ORIENTED_EDGE ( 'NONE', *, *, #16063, .T. ) ;
#23704=PLANE ( 'NONE',  #23383 ) ;
#23711=CARTESIAN_POINT ( 'NONE',  ( -7.730328572437709767, 4.608906612435681005, 21.50000000000000000 ) ) ;
#23715=AXIS2_PLACEMENT_3D ( 'NONE', #713, #260, #19289 ) ;
#23722=AXIS2_PLACEMENT_3D ( 'NONE', #5670, #5361, #22192 ) ;
#23727=VECTOR ( 'NONE', #21383, 1000.000000000000000 ) ;
#23740=AXIS2_PLACEMENT_3D ( 'NONE', #15336, #1004, #683 ) ;
#23743=ORIENTED_EDGE ( 'NONE', *, *, #25370, .F. ) ;
#23747=EDGE_LOOP ( 'NONE', ( #17517, #23773, #16893, #25574 ) ) ;
#23748=ORIENTED_EDGE ( 'NONE', *, *, #30735, .F. ) ;
#23753=DIRECTION ( 'NONE',  ( 0.000000000000000000, 1.132880637372608986E-16, -1.000000000000000000 ) ) ;
#23771=CIRCLE ( 'NONE', #2364, 0.7499999999999997780 ) ;
#23773=ORIENTED_EDGE ( 'NONE', *, *, #7295, .F. ) ;
#23777=DIRECTION ( 'NONE',  ( 0.000000000000000000, -1.132880637372608986E-16, 1.000000000000000000 ) ) ;
#23781=VECTOR ( 'NONE', #1500, 1000.000000000000000 ) ;
#23788=AXIS2_PLACEMENT_3D ( 'NONE', #18384, #16487, #23181 ) ;
#23795=DIRECTION ( 'NONE',  ( 0.000000000000000000, 1.000000000000000000, 0.000000000000000000 ) ) ;
#23800=DIRECTION ( 'NONE',  ( 0.000000000000000000, 0.000000000000000000, 1.000000000000000000 ) ) ;
#23806=CARTESIAN_POINT ( 'NONE',  ( -8.268028093133393597, -3.763133143576407047, -1.500000000000002220 ) ) ;
#23807=ORIENTED_EDGE ( 'NONE', *, *, #21361, .F. ) ;
#23811=DIRECTION ( 'NONE',  ( -0.000000000000000000, -0.000000000000000000, 1.000000000000000000 ) ) ;
#23821=CARTESIAN_POINT ( 'NONE',  ( 6.974883619896790954, 5.687793815610376669, -1.500000000000000888 ) ) ;
#23828=VERTEX_POINT ( 'NONE', #15006 ) ;
#23843=CARTESIAN_POINT ( 'NONE',  ( -3.993622308618940853, -8.159193615868383986, -1.500000000000002665 ) ) ;
#23846=LINE ( 'NONE', #7170, #1294 ) ;
#23851=DIRECTION ( 'NONE',  ( 0.000000000000000000, 0.000000000000000000, 1.000000000000000000 ) ) ;
#23860=EDGE_CURVE ( 'NONE', #18904, #28337, #7994, .T. ) ;
#23872=VERTEX_POINT ( 'NONE', #1456 ) ;
#23877=ORIENTED_EDGE ( 'NONE', *, *, #4387, .T. ) ;
#23892=DIRECTION ( 'NONE',  ( 3.642919299551291743E-14, 1.000000000000000000, 0.000000000000000000 ) ) ;
#23913=ORIENTED_EDGE ( 'NONE', *, *, #11084, .T. ) ;
#23924=EDGE_LOOP ( 'NONE', ( #20415, #12299, #4293, #3892 ) ) ;
#23933=AXIS2_PLACEMENT_3D ( 'NONE', #128, #26173, #14312 ) ;
#23939=CARTESIAN_POINT ( 'NONE',  ( -7.856594496258223259, -4.390207617113929039, -3.621320343559650379 ) ) ;
#23942=DIRECTION ( 'NONE',  ( -0.000000000000000000, 1.132880637372608986E-16, -1.000000000000000000 ) ) ;
#23951=CIRCLE ( 'NONE', #14490, 0.7500000000000006661 ) ;
#23966=EDGE_LOOP ( 'NONE', ( #9879, #10417 ) ) ;
#23967=ORIENTED_EDGE ( 'NONE', *, *, #8911, .T. ) ;
#23972=CIRCLE ( 'NONE', #8573, 15.00000000000003553 ) ;
#23978=ORIENTED_EDGE ( 'NONE', *, *, #10925, .T. ) ;
#23982=ORIENTED_EDGE ( 'NONE', *, *, #11266, .F. ) ;
#23989=DIRECTION ( 'NONE',  ( 0.000000000000000000, 1.000000000000000000, 0.000000000000000000 ) ) ;
#23994=CARTESIAN_POINT ( 'NONE',  ( -2.959227181723746547, 8.499586724479465616, -3.621320343559650379 ) ) ;
#24014=DIRECTION ( 'NONE',  ( 1.000000000000000000, 0.000000000000000000, 0.000000000000000000 ) ) ;
#24026=CARTESIAN_POINT ( 'NONE',  ( 0.000000000000000000, 15.00000000000003375, -87.50000000000000000 ) ) ;
#24039=LINE ( 'NONE', #14844, #10788 ) ;
#24047=DIRECTION ( 'NONE',  ( 0.000000000000000000, 1.000000000000000000, 1.193512090021232842E-16 ) ) ;
#24059=EDGE_CURVE ( 'NONE', #14477, #17470, #15452, .T. ) ;
#24062=AXIS2_PLACEMENT_3D ( 'NONE', #6131, #18150, #6596 ) ;
#24088=DIRECTION ( 'NONE',  ( 0.000000000000000000, 0.000000000000000000, 1.000000000000000000 ) ) ;
#24096=EDGE_CURVE ( 'NONE', #15632, #18015, #22913, .T. ) ;
#24101=EDGE_CURVE ( 'NONE', #26855, #9450, #12975, .T. ) ;
#24123=FACE_OUTER_BOUND ( 'NONE', #16220, .T. ) ;
#24136=VECTOR ( 'NONE', #17401, 1000.000000000000000 ) ;
#24146=DIRECTION ( 'NONE',  ( 0.000000000000000000, 0.000000000000000000, 1.000000000000000000 ) ) ;
#24154=CIRCLE ( 'NONE', #15199, 9.084132297865673777 ) ;
#24166=VERTEX_POINT ( 'NONE', #7030 ) ;
#24171=VERTEX_POINT ( 'NONE', #2659 ) ;
#24177=CIRCLE ( 'NONE', #8287, 0.7500000000000004441 ) ;
#24188=CARTESIAN_POINT ( 'NONE',  ( -9.062880100047301823, -0.6210184355499139830, 21.50000000000000000 ) ) ;
#24190=CARTESIAN_POINT ( 'NONE',  ( -1.438332125858111432, 8.884323311075791096, -3.621320343559650379 ) ) ;
#24192=DIRECTION ( 'NONE',  ( 0.000000000000000000, 0.000000000000000000, 1.000000000000000000 ) ) ;
#24200=ORIENTED_EDGE ( 'NONE', *, *, #21361, .T. ) ;
#24202=CARTESIAN_POINT ( 'NONE',  ( 0.000000000000000000, -2.435693370351110282E-15, 21.50000000000000355 ) ) ;
#24207=EDGE_CURVE ( 'NONE', #25420, #24589, #495, .T. ) ;
#24208=CIRCLE ( 'NONE', #12275, 0.7500000000000006661 ) ;
#24222=FACE_OUTER_BOUND ( 'NONE', #3909, .T. ) ;
#24224=CYLINDRICAL_SURFACE ( 'NONE', #21074, 0.7500000000000002220 ) ;
#24238=STYLED_ITEM('',(#30900),#2811);
#24240=EDGE_CURVE ( 'NONE', #699, #6203, #28400, .T. ) ;
#24247=DIRECTION ( 'NONE',  ( 0.000000000000000000, 0.000000000000000000, 1.000000000000000000 ) ) ;
#24249=ADVANCED_FACE ( 'NONE', ( #23054, #29951 ), #15740, .T. ) ;
#24260=ORIENTED_EDGE ( 'NONE', *, *, #21027, .T. ) ;
#24261=EDGE_CURVE ( 'NONE', #10933, #16535, #21931, .T. ) ;
#24263=EDGE_CURVE ( 'NONE', #23828, #30256, #23205, .T. ) ;
#24279=EDGE_CURVE ( 'NONE', #20523, #19687, #13967, .T. ) ;
#24282=CIRCLE ( 'NONE', #30727, 0.7500000000000006661 ) ;
#24283=CARTESIAN_POINT ( 'NONE',  ( 9.184850993605161750E-16, -7.500000000000018652, -1.500000000000002220 ) ) ;
#24285=DIRECTION ( 'NONE',  ( 1.000000000000000000, 0.000000000000000000, 0.000000000000000000 ) ) ;
#24308=AXIS2_PLACEMENT_3D ( 'NONE', #9515, #4829, #14345 ) ;
#24309=CARTESIAN_POINT ( 'NONE',  ( -8.413215745754975217, 3.196529495465474380, -3.621320343559650379 ) ) ;
#24313=EDGE_CURVE ( 'NONE', #1903, #9741, #28419, .T. ) ;
#24318=ORIENTED_EDGE ( 'NONE', *, *, #26386, .F. ) ;
#24322=FACE_OUTER_BOUND ( 'NONE', #9081, .T. ) ;
#24327=ORIENTED_EDGE ( 'NONE', *, *, #22763, .F. ) ;
#24330=DIRECTION ( 'NONE',  ( 1.000000000000000000, 0.000000000000000000, 0.000000000000000000 ) ) ;
#24335=ORIENTED_EDGE ( 'NONE', *, *, #18316, .F. ) ;
#24342=DIRECTION ( 'NONE',  ( 0.000000000000000000, -1.132880637372608986E-16, 1.000000000000000000 ) ) ;
#24347=ORIENTED_EDGE ( 'NONE', *, *, #21757, .F. ) ;
#24349=CARTESIAN_POINT ( 'NONE',  ( -8.303920738747237351, -3.683253992019804191, 13.22130136205108819 ) ) ;
#24367=PLANE ( 'NONE',  #21280 ) ;
#24368=ORIENTED_EDGE ( 'NONE', *, *, #8447, .T. ) ;
#24380=DIRECTION ( 'NONE',  ( 1.000000000000000000, 0.000000000000000000, 0.000000000000000000 ) ) ;
#24381=CARTESIAN_POINT ( 'NONE',  ( 7.341751895053238108, -5.349779314757616255, 21.50000000000000000 ) ) ;
#24383=ORIENTED_EDGE ( 'NONE', *, *, #14898, .T. ) ;
#24427=CARTESIAN_POINT ( 'NONE',  ( -8.884323311075783991, -1.438332125858144295, -3.621320343559650379 ) ) ;
#24437=EDGE_CURVE ( 'NONE', #19662, #25948, #28375, .T. ) ;
#24439=EDGE_CURVE ( 'NONE', #11684, #6919, #30419, .T. ) ;
#24456=EDGE_CURVE ( 'NONE', #14124, #11549, #280, .T. ) ;
#24464=FACE_OUTER_BOUND ( 'NONE', #22294, .T. ) ;
#24466=VERTEX_POINT ( 'NONE', #25876 ) ;
#24476=CARTESIAN_POINT ( 'NONE',  ( 8.499586724479435418, 2.959227181723830036, 21.50000000000000000 ) ) ;
#24481=AXIS2_PLACEMENT_3D ( 'NONE', #23034, #15566, #13408 ) ;
#24495=DIRECTION ( 'NONE',  ( 0.000000000000000000, 1.000000000000000000, 0.000000000000000000 ) ) ;
#24517=ORIENTED_EDGE ( 'NONE', *, *, #1623, .T. ) ;
#24526=ADVANCED_FACE ( 'NONE', ( #10721 ), #5587, .F. ) ;
#24530=FACE_OUTER_BOUND ( 'NONE', #13178, .T. ) ;
#24540=FACE_OUTER_BOUND ( 'NONE', #28969, .T. ) ;
#24548=ORIENTED_EDGE ( 'NONE', *, *, #24261, .F. ) ;
#24563=ORIENTED_EDGE ( 'NONE', *, *, #18731, .F. ) ;
#24587=VECTOR ( 'NONE', #26283, 1000.000000000000000 ) ;
#24589=VERTEX_POINT ( 'NONE', #10103 ) ;
#24608=EDGE_CURVE ( 'NONE', #14972, #28030, #5508, .T. ) ;
#24630=AXIS2_PLACEMENT_3D ( 'NONE', #16047, #1409, #9037 ) ;
#24634=EDGE_CURVE ( 'NONE', #27497, #10212, #22717, .T. ) ;
#24663=EDGE_CURVE ( 'NONE', #14718, #11152, #17472, .T. ) ;
#24666=EDGE_CURVE ( 'NONE', #19689, #30824, #27468, .T. ) ;
#24672=ORIENTED_EDGE ( 'NONE', *, *, #28987, .F. ) ;
#24676=CIRCLE ( 'NONE', #4745, 0.7500000000000006661 ) ;
#24695=AXIS2_PLACEMENT_3D ( 'NONE', #26292, #19123, #28490 ) ;
#24698=AXIS2_PLACEMENT_3D ( 'NONE', #18091, #29949, #20270 ) ;
#24699=DIRECTION ( 'NONE',  ( 0.000000000000000000, 0.000000000000000000, 1.000000000000000000 ) ) ;
#24700=EDGE_LOOP ( 'NONE', ( #23160, #26141, #15242 ) ) ;
#24709=AXIS2_PLACEMENT_3D ( 'NONE', #6021, #26941, #1193 ) ;
#24712=CARTESIAN_POINT ( 'NONE',  ( 0.000000000000000000, 7.500000000000000000, -1.500000000000000888 ) ) ;
#24715=EDGE_LOOP ( 'NONE', ( #4605, #796, #25712, #8598, #20360, #17989, #4128, #22226, #17616, #15031, #14955, #6516, #17316, #7190, #27882, #13620, #11879, #6705, #10669, #15741, #15288, #30582, #23967, #18688, #27115, #13236, #23703, #29905, #21672, #18718, #23913, #26714, #17746, #29629, #6393, #11746, #29745, #15737, #22125, #25645, #18485, #6074, #8343, #10018, #13029, #23522, #19306, #1587, #23387, #14152, #27933, #21519, #17898, #25646, #11793, #3927, #13306, #853, #11857, #22673, #21804, #19309, #2147, #21568, #12063, #22396, #30136, #10206, #1011, #3592, #507, #25817, #20300, #10381, #23877, #15897 ) ) ;
#24719=DIRECTION ( 'NONE',  ( 1.000000000000000000, 0.000000000000000000, 0.000000000000000000 ) ) ;
#24728=CARTESIAN_POINT ( 'NONE',  ( 2.270234684139676773, -8.795879380940572645, 21.50000000000000000 ) ) ;
#24729=CIRCLE ( 'NONE', #8800, 9.084132297865673777 ) ;
#24734=CARTESIAN_POINT ( 'NONE',  ( 0.000000000000000000, 12.18947652193946851, 29.43090101791767665 ) ) ;
#24738=AXIS2_PLACEMENT_3D ( 'NONE', #26390, #5015, #11724 ) ;
#24739=ORIENTED_EDGE ( 'NONE', *, *, #2706, .T. ) ;
#24744=DIRECTION ( 'NONE',  ( 0.000000000000000000, 1.000000000000000000, 0.000000000000000000 ) ) ;
#24775=CIRCLE ( 'NONE', #5860, 9.084132297865673777 ) ;
#24778=AXIS2_PLACEMENT_3D ( 'NONE', #11324, #21269, #20821 ) ;
#24785=EDGE_CURVE ( 'NONE', #1968, #19482, #12511, .T. ) ;
#24799=ADVANCED_FACE ( 'NONE', ( #24464 ), #7628, .F. ) ;
#24805=CYLINDRICAL_SURFACE ( 'NONE', #21846, 0.7500000000000006661 ) ;
#24815=CARTESIAN_POINT ( 'NONE',  ( -7.392982946727045146, 5.278755796068742789, 21.50000000000000000 ) ) ;
#24817=EDGE_CURVE ( 'NONE', #18115, #23298, #25470, .T. ) ;
#24820=LINE ( 'NONE', #3458, #22762 ) ;
#24828=EDGE_CURVE ( 'NONE', #3530, #28571, #9036, .T. ) ;
#24847=CARTESIAN_POINT ( 'NONE',  ( -8.752572334588105463, 2.431858781452820306, 13.22130136205108819 ) ) ;
#24853=DIRECTION ( 'NONE',  ( -0.000000000000000000, -0.000000000000000000, 1.000000000000000000 ) ) ;
#24856=VECTOR ( 'NONE', #1124, 1000.000000000000000 ) ;
#24858=DIRECTION ( 'NONE',  ( 0.000000000000000000, 0.000000000000000000, 1.000000000000000000 ) ) ;
#24864=CIRCLE ( 'NONE', #10911, 0.7500000000000006661 ) ;
#24871=AXIS2_PLACEMENT_3D ( 'NONE', #2068, #16567, #11589 ) ;
#24872=CARTESIAN_POINT ( 'NONE',  ( 3.196529495465388226, 8.413215745755008967, -3.621320343559650379 ) ) ;
#24874=ORIENTED_EDGE ( 'NONE', *, *, #21033, .T. ) ;
#24893=PLANE ( 'NONE',  #4839 ) ;
#24896=DIRECTION ( 'NONE',  ( 0.000000000000000000, 1.000000000000000000, 1.193512090021232842E-16 ) ) ;
#24900=DIRECTION ( 'NONE',  ( 1.000000000000000000, 0.000000000000000000, 0.000000000000000000 ) ) ;
#24909=FACE_OUTER_BOUND ( 'NONE', #1638, .T. ) ;
#24911=AXIS2_PLACEMENT_3D ( 'NONE', #23614, #11778, #4148 ) ;
#24913=CARTESIAN_POINT ( 'NONE',  ( -4.608906612435655248, -7.730328572437724866, -3.621320343559650379 ) ) ;
#24924=CARTESIAN_POINT ( 'NONE',  ( 6.364020599487795415, -6.482337650448428690, -1.500000000000002442 ) ) ;
#24937=CARTESIAN_POINT ( 'NONE',  ( -3.858906612435654804, -7.730328572437724866, 21.50000000000000000 ) ) ;
#24945=AXIS2_PLACEMENT_3D ( 'NONE', #22878, #1673, #11038 ) ;
#24949=DIRECTION ( 'NONE',  ( 0.000000000000000000, 1.000000000000000000, 0.000000000000000000 ) ) ;
#24980=CARTESIAN_POINT ( 'NONE',  ( -8.999114229549592281, 0.1262659238205133538, -3.621320343559650379 ) ) ;
#24991=EDGE_CURVE ( 'NONE', #23872, #11382, #4041, .T. ) ;
#24999=CIRCLE ( 'NONE', #3072, 0.7500000000000006661 ) ;
#25006=CYLINDRICAL_SURFACE ( 'NONE', #24062, 0.7499999999999997780 ) ;
#25008=ORIENTED_EDGE ( 'NONE', *, *, #13221, .T. ) ;
#25039=CIRCLE ( 'NONE', #11590, 9.084132297865673777 ) ;
#25053=ORIENTED_EDGE ( 'NONE', *, *, #3805, .F. ) ;
#25071=CARTESIAN_POINT ( 'NONE',  ( 0.6210184355499435149, -9.062880100047300047, -1.500000000000002887 ) ) ;
#25072=VECTOR ( 'NONE', #11918, 1000.000000000000000 ) ;
#25081=DIRECTION ( 'NONE',  ( 1.000000000000000000, 0.000000000000000000, 0.000000000000000000 ) ) ;
#25091=CARTESIAN_POINT ( 'NONE',  ( -6.812559277181930106, 5.881244434206302607, 21.50000000000000000 ) ) ;
#25100=LINE ( 'NONE', #3743, #5693 ) ;
#25103=ORIENTED_EDGE ( 'NONE', *, *, #28683, .F. ) ;
#25108=VERTEX_POINT ( 'NONE', #26629 ) ;
#25114=ORIENTED_EDGE ( 'NONE', *, *, #24785, .T. ) ;
#25127=EDGE_LOOP ( 'NONE', ( #23748, #15134, #29038, #19546 ) ) ;
#25133=CARTESIAN_POINT ( 'NONE',  ( 8.303920738747214259, 3.683253992019856149, 21.50000000000000000 ) ) ;
#25134=CARTESIAN_POINT ( 'NONE',  ( 9.184850993605159777E-16, -7.500000000000015099, -16.50000000000000000 ) ) ;
#25137=CARTESIAN_POINT ( 'NONE',  ( 0.000000000000000000, -2.775557561562891351E-14, 157.4999999999999716 ) ) ;
#25138=CARTESIAN_POINT ( 'NONE',  ( -8.817355867515827228, -2.185336383880175593, 21.50000000000000000 ) ) ;
#25139=DIRECTION ( 'NONE',  ( 0.000000000000000000, 0.000000000000000000, 1.000000000000000000 ) ) ;
#25151=DIRECTION ( 'NONE',  ( -0.000000000000000000, -0.000000000000000000, 1.000000000000000000 ) ) ;
#25155=VERTEX_POINT ( 'NONE', #880 ) ;
#25169=EDGE_CURVE ( 'NONE', #18098, #20761, #1555, .T. ) ;
#25195=ADVANCED_FACE ( 'NONE', ( #22401 ), #13364, .F. ) ;
#25204=CARTESIAN_POINT ( 'NONE',  ( 0.000000000000000000, 1.699320956058915452E-16, -1.500000000000001776 ) ) ;
#25206=DIRECTION ( 'NONE',  ( 1.000000000000000000, 0.000000000000000000, 0.000000000000000000 ) ) ;
#25212=CIRCLE ( 'NONE', #22228, 9.084132297865673777 ) ;
#25218=LINE ( 'NONE', #26248, #13280 ) ;
#25222=ORIENTED_EDGE ( 'NONE', *, *, #26131, .F. ) ;
#25231=ADVANCED_FACE ( 'NONE', ( #1508 ), #13202, .F. ) ;
#25240=EDGE_CURVE ( 'NONE', #15826, #26641, #17491, .T. ) ;
#25252=CIRCLE ( 'NONE', #18291, 0.7500000000000007772 ) ;
#25255=MECHANICAL_DESIGN_GEOMETRIC_PRESENTATION_REPRESENTATION('',(#24238),#26673);
#25260=DIRECTION ( 'NONE',  ( -0.000000000000000000, 1.132880637372608986E-16, -1.000000000000000000 ) ) ;
#25261=ORIENTED_EDGE ( 'NONE', *, *, #4387, .F. ) ;
#25267=ORIENTED_EDGE ( 'NONE', *, *, #13934, .T. ) ;
#25269=AXIS2_PLACEMENT_3D ( 'NONE', #28927, #17063, #10051 ) ;
#25282=DIRECTION ( 'NONE',  ( -0.000000000000000000, 1.132880637372608986E-16, -1.000000000000000000 ) ) ;
#25292=DIRECTION ( 'NONE',  ( -0.000000000000000000, 1.132880637372608986E-16, -1.000000000000000000 ) ) ;
#25295=DIRECTION ( 'NONE',  ( 0.000000000000000000, 0.000000000000000000, 1.000000000000000000 ) ) ;
#25302=DIRECTION ( 'NONE',  ( -0.000000000000000000, 1.132880637372608986E-16, -1.000000000000000000 ) ) ;
#25321=VECTOR ( 'NONE', #18752, 1000.000000000000000 ) ;
#25334=DIRECTION ( 'NONE',  ( 0.000000000000000000, 0.000000000000000000, 1.000000000000000000 ) ) ;
#25347=DIRECTION ( 'NONE',  ( 0.000000000000000000, -1.132880637372608986E-16, 1.000000000000000000 ) ) ;
#25358=VECTOR ( 'NONE', #22830, 1000.000000000000000 ) ;
#25367=ORIENTED_EDGE ( 'NONE', *, *, #10232, .F. ) ;
#25368=EDGE_LOOP ( 'NONE', ( #14813, #9823, #21848 ) ) ;
#25370=EDGE_CURVE ( 'NONE', #19662, #30243, #18030, .T. ) ;
#25374=ORIENTED_EDGE ( 'NONE', *, *, #15692, .T. ) ;
#25380=ORIENTED_EDGE ( 'NONE', *, *, #15695, .T. ) ;
#25392=DIRECTION ( 'NONE',  ( 1.000000000000000000, 0.000000000000000000, 0.000000000000000000 ) ) ;
#25407=CIRCLE ( 'NONE', #11962, 9.084132297865673777 ) ;
#25410=EDGE_CURVE ( 'NONE', #11295, #26463, #23972, .T. ) ;
#25420=VERTEX_POINT ( 'NONE', #25518 ) ;
#25442=ADVANCED_FACE ( 'NONE', ( #9127 ), #18647, .T. ) ;
#25466=VERTEX_POINT ( 'NONE', #6947 ) ;
#25470=CIRCLE ( 'NONE', #1063, 0.7500000000000002220 ) ;
#25486=CYLINDRICAL_SURFACE ( 'NONE', #15557, 0.7499999999999997780 ) ;
#25497=VERTEX_POINT ( 'NONE', #14098 ) ;
#25510=CARTESIAN_POINT ( 'NONE',  ( 1.836970198721033928E-15, -15.00000000000003375, -87.50000000000000000 ) ) ;
#25513=DIRECTION ( 'NONE',  ( -0.000000000000000000, 1.132880637372608986E-16, -1.000000000000000000 ) ) ;
#25518=CARTESIAN_POINT ( 'NONE',  ( 7.538175180318423152, 5.069257791428403159, 21.50000000000000000 ) ) ;
#25520=VECTOR ( 'NONE', #12197, 1000.000000000000000 ) ;
#25538=CIRCLE ( 'NONE', #14579, 10.00000000000003730 ) ;
#25542=CARTESIAN_POINT ( 'NONE',  ( 4.390207617113956573, -7.856594496258208160, -3.621320343559650379 ) ) ;
#25549=CARTESIAN_POINT ( 'NONE',  ( 9.033033306777456417, -0.9621688436939737077, -1.500000000000001998 ) ) ;
#25551=CARTESIAN_POINT ( 'NONE',  ( 3.993622308618882677, 8.159193615868414184, -1.500000000000000888 ) ) ;
#25554=ORIENTED_EDGE ( 'NONE', *, *, #25987, .T. ) ;
#25560=CIRCLE ( 'NONE', #28537, 0.7500000000000006661 ) ;
#25564=EDGE_CURVE ( 'NONE', #8444, #2547, #19509, .T. ) ;
#25570=CARTESIAN_POINT ( 'NONE',  ( -7.106594496258223259, -4.390207617113929039, 21.50000000000000000 ) ) ;
#25571=DIRECTION ( 'NONE',  ( 0.000000000000000000, 1.000000000000000000, 1.132880637372608986E-16 ) ) ;
#25574=ORIENTED_EDGE ( 'NONE', *, *, #25370, .T. ) ;
#25579=EDGE_CURVE ( 'NONE', #5755, #17047, #8489, .T. ) ;
#25584=DIRECTION ( 'NONE',  ( 0.000000000000000000, 1.132880637372608986E-16, -1.000000000000000000 ) ) ;
#25589=ORIENTED_EDGE ( 'NONE', *, *, #20028, .F. ) ;
#25595=ORIENTED_EDGE ( 'NONE', *, *, #12446, .T. ) ;
#25600=CIRCLE ( 'NONE', #17145, 15.00000000000003375 ) ;
#25603=ADVANCED_FACE ( 'NONE', ( #26214 ), #2519, .F. ) ;
#25620=DIRECTION ( 'NONE',  ( 0.000000000000000000, -1.132880637372608986E-16, 1.000000000000000000 ) ) ;
#25645=ORIENTED_EDGE ( 'NONE', *, *, #4473, .T. ) ;
#25646=ORIENTED_EDGE ( 'NONE', *, *, #24991, .F. ) ;
#25648=DIRECTION ( 'NONE',  ( 0.000000000000000000, 1.000000000000000000, 0.000000000000000000 ) ) ;
#25655=LINE ( 'NONE', #520, #5380 ) ;
#25660=DIRECTION ( 'NONE',  ( 1.000000000000000000, 0.000000000000000000, 0.000000000000000000 ) ) ;
#25689=DIRECTION ( 'NONE',  ( 1.000000000000000000, 0.000000000000000000, 0.000000000000000000 ) ) ;
#25690=EDGE_LOOP ( 'NONE', ( #4723, #8252, #6543, #398 ) ) ;
#25700=DIRECTION ( 'NONE',  ( 1.000000000000000000, 0.000000000000000000, 0.000000000000000000 ) ) ;
#25704=ORIENTED_EDGE ( 'NONE', *, *, #23860, .F. ) ;
#25709=CIRCLE ( 'NONE', #18715, 0.7500000000000002220 ) ;
#25712=ORIENTED_EDGE ( 'NONE', *, *, #29471, .T. ) ;
#25725=AXIS2_PLACEMENT_3D ( 'NONE', #27859, #18497, #2095 ) ;
#25732=ORIENTED_EDGE ( 'NONE', *, *, #4434, .F. ) ;
#25736=DIRECTION ( 'NONE',  ( 1.000000000000000000, 0.000000000000000000, 0.000000000000000000 ) ) ;
#25761=AXIS2_PLACEMENT_3D ( 'NONE', #28392, #16526, #26192 ) ;
#25764=EDGE_CURVE ( 'NONE', #27309, #14218, #5085, .T. ) ;
#25765=CLOSED_SHELL ( 'NONE', ( #765, #25785, #14883, #20758, #25231, #449, #24526, #5988, #18199, #5737, #28659, #26554, #1720, #1999, #3504, #25603, #5631, #30173, #28835, #28478, #13436, #2934, #3668, #20214, #3887, #25962, #6348, #24249, #16625, #1950, #8487, #7830, #25442, #14275, #1214, #5352, #29076, #1762, #5633, #2628, #26675, #25195, #22152, #1451, #9929, #8069, #12075, #26328, #23312, #28452, #16031, #12623, #22516, #29796, #6545, #13392, #25958, #5026, #15835, #20096, #4397, #22812, #22514, #6677, #7318, #15102, #14541, #16022, #27922, #6011, #9697, #2718, #16856, #28667, #5991, #28098, #5724, #1159, #22062, #19308, #12454, #795, #28630, #11686, #14002, #9999, #10563, #25843, #6368, #3279, #14196, #26157, #24799, #30065, #28516, #28644, #30682, #23099, #1228, #22335, #13744, #16191, #13778, #1925, #5001, #6724, #20833, #1944, #11441, #27482, #8503, #20601 ) ) ;
#25766=DIRECTION ( 'NONE',  ( 1.000000000000000000, 0.000000000000000000, 0.000000000000000000 ) ) ;
#25767=EDGE_CURVE ( 'NONE', #1665, #17197, #1104, .T. ) ;
#25768=DIRECTION ( 'NONE',  ( 1.000000000000000000, 0.000000000000000000, 0.000000000000000000 ) ) ;
#25781=EDGE_CURVE ( 'NONE', #17742, #1033, #17033, .T. ) ;
#25785=ADVANCED_FACE ( 'NONE', ( #7662 ), #28880, .F. ) ;
#25798=AXIS2_PLACEMENT_3D ( 'NONE', #13691, #23023, #16329 ) ;
#25801=AXIS2_PLACEMENT_3D ( 'NONE', #20765, #2052, #20477 ) ;
#25809=CIRCLE ( 'NONE', #12365, 9.084132297865673777 ) ;
#25817=ORIENTED_EDGE ( 'NONE', *, *, #26386, .T. ) ;
#25822=DIRECTION ( 'NONE',  ( -0.000000000000000000, 1.132880637372608986E-16, -1.000000000000000000 ) ) ;
#25828=VERTEX_POINT ( 'NONE', #18062 ) ;
#25834=VECTOR ( 'NONE', #25513, 1000.000000000000000 ) ;
#25836=AXIS2_PLACEMENT_3D ( 'NONE', #14290, #28505, #14000 ) ;
#25843=ADVANCED_FACE ( 'NONE', ( #11191 ), #15873, .F. ) ;
#25844=VECTOR ( 'NONE', #13529, 1000.000000000000000 ) ;
#25845=DIRECTION ( 'NONE',  ( 0.000000000000000000, 1.000000000000000000, 0.000000000000000000 ) ) ;
#25847=ORIENTED_EDGE ( 'NONE', *, *, #21943, .F. ) ;
#25852=CARTESIAN_POINT ( 'NONE',  ( 6.812559277181973627, -5.881244434206257310, 21.50000000000000000 ) ) ;
#25853=CARTESIAN_POINT ( 'NONE',  ( 0.000000000000000000, 0.000000000000000000, -87.50000000000000000 ) ) ;
#25856=CIRCLE ( 'NONE', #15910, 0.7500000000000011102 ) ;
#25860=CARTESIAN_POINT ( 'NONE',  ( 5.278755796068665518, 7.392982946727100213, 21.50000000000000000 ) ) ;
#25863=VECTOR ( 'NONE', #28551, 1000.000000000000000 ) ;
#25872=EDGE_LOOP ( 'NONE', ( #14590, #1922 ) ) ;
#25873=DIRECTION ( 'NONE',  ( 0.000000000000000000, 1.000000000000000000, 1.193512090021232842E-16 ) ) ;
#25876=CARTESIAN_POINT ( 'NONE',  ( -0.9370274472974918778, -8.840471615930066918, 21.50000000000000000 ) ) ;
#25893=ORIENTED_EDGE ( 'NONE', *, *, #16744, .F. ) ;
#25896=PLANE ( 'NONE',  #2662 ) ;
#25901=FACE_OUTER_BOUND ( 'NONE', #23924, .T. ) ;
#25908=CARTESIAN_POINT ( 'NONE',  ( 0.000000000000000000, 1.699320956058915452E-16, -1.500000000000001776 ) ) ;
#25921=CARTESIAN_POINT ( 'NONE',  ( -4.608906612435655248, -7.730328572437724866, 21.50000000000000000 ) ) ;
#25924=ORIENTED_EDGE ( 'NONE', *, *, #7106, .F. ) ;
#25926=CARTESIAN_POINT ( 'NONE',  ( 0.000000000000000000, 1.699320956058915452E-16, -1.500000000000001776 ) ) ;
#25927=DIRECTION ( 'NONE',  ( -8.673617379884027583E-16, 1.000000000000000000, 0.000000000000000000 ) ) ;
#25948=VERTEX_POINT ( 'NONE', #13693 ) ;
#25949=EDGE_CURVE ( 'NONE', #19691, #1661, #594, .T. ) ;
#25955=EDGE_CURVE ( 'NONE', #28009, #15594, #3083, .T. ) ;
#25958=ADVANCED_FACE ( 'NONE', ( #23632 ), #9302, .F. ) ;
#25962=ADVANCED_FACE ( 'NONE', ( #26139 ), #28496, .T. ) ;
#25972=DIRECTION ( 'NONE',  ( -0.000000000000000000, -0.000000000000000000, 1.000000000000000000 ) ) ;
#25987=EDGE_CURVE ( 'NONE', #4497, #7702, #4585, .T. ) ;
#25991=EDGE_CURVE ( 'NONE', #28059, #30853, #7126, .T. ) ;
#25993=AXIS2_PLACEMENT_3D ( 'NONE', #11505, #7589, #14126 ) ;
#26000=DIRECTION ( 'NONE',  ( -0.000000000000000000, -0.000000000000000000, 1.000000000000000000 ) ) ;
#26020=VERTEX_POINT ( 'NONE', #2598 ) ;
#26023=AXIS2_PLACEMENT_3D ( 'NONE', #30043, #8684, #16609 ) ;
#26040=DIRECTION ( 'NONE',  ( 0.000000000000000000, -1.132880637372608986E-16, 1.000000000000000000 ) ) ;
#26044=VERTEX_POINT ( 'NONE', #16638 ) ;
#26058=ORIENTED_EDGE ( 'NONE', *, *, #12406, .F. ) ;
#26062=CARTESIAN_POINT ( 'NONE',  ( -5.687793815610304726, 6.974883619896852238, 21.50000000000000000 ) ) ;
#26068=CYLINDRICAL_SURFACE ( 'NONE', #13515, 0.7500000000000006661 ) ;
#26070=CARTESIAN_POINT ( 'NONE',  ( -6.482337650448453559, -6.364020599487773211, -1.500000000000002442 ) ) ;
#26095=ORIENTED_EDGE ( 'NONE', *, *, #7568, .F. ) ;
#26096=ORIENTED_EDGE ( 'NONE', *, *, #12893, .F. ) ;
#26097=CARTESIAN_POINT ( 'NONE',  ( -6.062559277181930106, 5.881244434206302607, -3.621320343559650379 ) ) ;
#26099=ORIENTED_EDGE ( 'NONE', *, *, #13806, .F. ) ;
#26103=CARTESIAN_POINT ( 'NONE',  ( -5.687793815610304726, 6.974883619896852238, 21.50000000000000000 ) ) ;
#26131=EDGE_CURVE ( 'NONE', #30824, #16597, #26496, .T. ) ;
#26139=FACE_OUTER_BOUND ( 'NONE', #19752, .T. ) ;
#26141=ORIENTED_EDGE ( 'NONE', *, *, #1983, .F. ) ;
#26157=ADVANCED_FACE ( 'NONE', ( #27392 ), #26774, .F. ) ;
#26159=LINE ( 'NONE', #9482, #27529 ) ;
#26173=DIRECTION ( 'NONE',  ( 0.000000000000000000, 0.000000000000000000, 1.000000000000000000 ) ) ;
#26176=ORIENTED_EDGE ( 'NONE', *, *, #22337, .T. ) ;
#26185=CIRCLE ( 'NONE', #4767, 9.084132297865673777 ) ;
#26191=DIRECTION ( 'NONE',  ( 0.000000000000000000, 1.000000000000000000, 0.000000000000000000 ) ) ;
#26192=DIRECTION ( 'NONE',  ( 1.000000000000000000, 0.000000000000000000, -0.000000000000000000 ) ) ;
#26200=CARTESIAN_POINT ( 'NONE',  ( -0.9621688436940063482, -9.033033306777452864, -1.500000000000002887 ) ) ;
#26206=DIRECTION ( 'NONE',  ( 0.000000000000000000, 0.000000000000000000, 1.000000000000000000 ) ) ;
#26210=EDGE_CURVE ( 'NONE', #27497, #23872, #27958, .T. ) ;
#26214=FACE_OUTER_BOUND ( 'NONE', #15925, .T. ) ;
#26215=ORIENTED_EDGE ( 'NONE', *, *, #4227, .T. ) ;
#26231=AXIS2_PLACEMENT_3D ( 'NONE', #23711, #21067, #25766 ) ;
#26235=DIRECTION ( 'NONE',  ( -0.000000000000000000, -0.000000000000000000, 1.000000000000000000 ) ) ;
#26248=CARTESIAN_POINT ( 'NONE',  ( -0.6883321258581104329, 8.884323311075791096, -3.621320343559650379 ) ) ;
#26257=DIRECTION ( 'NONE',  ( 0.000000000000000000, 0.000000000000000000, 1.000000000000000000 ) ) ;
#26269=DIRECTION ( 'NONE',  ( -0.000000000000000000, 1.132880637372608986E-16, -1.000000000000000000 ) ) ;
#26280=CARTESIAN_POINT ( 'NONE',  ( -4.390207617113899730, 7.856594496258241023, 21.50000000000000000 ) ) ;
#26283=DIRECTION ( 'NONE',  ( -0.000000000000000000, 1.132880637372608986E-16, -1.000000000000000000 ) ) ;
#26292=CARTESIAN_POINT ( 'NONE',  ( -2.959227181723746547, 8.499586724479465616, 21.50000000000000000 ) ) ;
#26293=AXIS2_PLACEMENT_3D ( 'NONE', #1344, #1194, #15679 ) ;
#26310=EDGE_CURVE ( 'NONE', #8541, #386, #7082, .T. ) ;
#26319=AXIS2_PLACEMENT_3D ( 'NONE', #9977, #24146, #28850 ) ;
#26326=AXIS2_PLACEMENT_3D ( 'NONE', #12345, #14823, #163 ) ;
#26327=DIRECTION ( 'NONE',  ( 1.000000000000000000, 0.000000000000000000, -0.000000000000000000 ) ) ;
#26328=ADVANCED_FACE ( 'NONE', ( #24530 ), #5823, .F. ) ;
#26339=EDGE_CURVE ( 'NONE', #9285, #30374, #11077, .T. ) ;
#26340=CIRCLE ( 'NONE', #2351, 0.7500000000000006661 ) ;
#26344=EDGE_CURVE ( 'NONE', #16202, #11358, #23951, .T. ) ;
#26354=CARTESIAN_POINT ( 'NONE',  ( 1.836970198721033928E-15, -15.00000000000004796, 29.43090101791767665 ) ) ;
#26365=CIRCLE ( 'NONE', #5929, 9.084132297865673777 ) ;
#26386=EDGE_CURVE ( 'NONE', #14711, #27939, #20471, .T. ) ;
#26388=DIRECTION ( 'NONE',  ( 1.000000000000000000, 0.000000000000000000, 0.000000000000000000 ) ) ;
#26390=CARTESIAN_POINT ( 'NONE',  ( 0.000000000000000000, -2.435693370351110282E-15, 21.50000000000000355 ) ) ;
#26414=DIRECTION ( 'NONE',  ( 1.000000000000000000, 0.000000000000000000, 0.000000000000000000 ) ) ;
#26416=ORIENTED_EDGE ( 'NONE', *, *, #20033, .T. ) ;
#26420=ORIENTED_EDGE ( 'NONE', *, *, #25579, .F. ) ;
#26463=VERTEX_POINT ( 'NONE', #27506 ) ;
#26467=CARTESIAN_POINT ( 'NONE',  ( -8.840471615930058036, 1.687027447297517080, -1.500000000000001776 ) ) ;
#26468=DIRECTION ( 'NONE',  ( 1.000000000000000000, 0.000000000000000000, 0.000000000000000000 ) ) ;
#26480=ORIENTED_EDGE ( 'NONE', *, *, #26210, .F. ) ;
#26483=DIRECTION ( 'NONE',  ( 0.000000000000000000, 0.000000000000000000, 1.000000000000000000 ) ) ;
#26484=ORIENTED_EDGE ( 'NONE', *, *, #24666, .T. ) ;
#26491=AXIS2_PLACEMENT_3D ( 'NONE', #27900, #6523, #22580 ) ;
#26496=CIRCLE ( 'NONE', #12554, 9.084132297865673777 ) ;
#26509=APPLICATION_CONTEXT ( 'automotive_design' ) ;
#26524=CARTESIAN_POINT ( 'NONE',  ( 0.000000000000000000, -2.435693370351110282E-15, 21.50000000000000355 ) ) ;
#26525=VERTEX_POINT ( 'NONE', #11124 ) ;
#26528=ORIENTED_EDGE ( 'NONE', *, *, #2529, .F. ) ;
#26534=VECTOR ( 'NONE', #24342, 1000.000000000000000 ) ;
#26539=CARTESIAN_POINT ( 'NONE',  ( 0.000000000000000000, -7.422978769709303177E-15, 65.52304386563415051 ) ) ;
#26554=ADVANCED_FACE ( 'NONE', ( #30444 ), #26068, .F. ) ;
#26556=CARTESIAN_POINT ( 'NONE',  ( -0.8762659238204844048, -8.999114229549588728, -1.500000000000002665 ) ) ;
#26562=EDGE_CURVE ( 'NONE', #14218, #20523, #168, .T. ) ;
#26570=ORIENTED_EDGE ( 'NONE', *, *, #8098, .T. ) ;
#26571=CIRCLE ( 'NONE', #16606, 0.7500000000000006661 ) ;
#26572=ORIENTED_EDGE ( 'NONE', *, *, #29930, .F. ) ;
#26617=DIRECTION ( 'NONE',  ( 0.000000000000000000, 1.132880637372608986E-16, -1.000000000000000000 ) ) ;
#26618=EDGE_CURVE ( 'NONE', #34, #16268, #18082, .T. ) ;
#26629=CARTESIAN_POINT ( 'NONE',  ( 6.543385983536347261, 6.301234758012619785, -1.500000000000001110 ) ) ;
#26641=VERTEX_POINT ( 'NONE', #2051 ) ;
#26658=ORIENTED_EDGE ( 'NONE', *, *, #12059, .F. ) ;
#26673=( GEOMETRIC_REPRESENTATION_CONTEXT ( 3 ) GLOBAL_UNCERTAINTY_ASSIGNED_CONTEXT ( ( #28562 ) ) GLOBAL_UNIT_ASSIGNED_CONTEXT ( ( #18067, #12766, #29460 ) ) REPRESENTATION_CONTEXT ( 'NONE', 'WORKASPACE' ) );
#26674=DIRECTION ( 'NONE',  ( 0.000000000000000000, 1.000000000000000000, 1.193512090021232842E-16 ) ) ;
#26675=ADVANCED_FACE ( 'NONE', ( #9231 ), #18746, .F. ) ;
#26685=AXIS2_PLACEMENT_3D ( 'NONE', #17655, #798, #22013 ) ;
#26708=CIRCLE ( 'NONE', #30676, 0.7500000000000006661 ) ;
#26710=CARTESIAN_POINT ( 'NONE',  ( -2.209227181723746103, 8.499586724479465616, -1.500000000000000888 ) ) ;
#26714=ORIENTED_EDGE ( 'NONE', *, *, #10935, .T. ) ;
#26727=EDGE_CURVE ( 'NONE', #25497, #14711, #12812, .T. ) ;
#26728=CARTESIAN_POINT ( 'NONE',  ( -8.413215745754975217, 3.196529495465474380, -1.500000000000001332 ) ) ;
#26740=VECTOR ( 'NONE', #7280, 1000.000000000000000 ) ;
#26749=AXIS2_PLACEMENT_3D ( 'NONE', #20335, #10511, #19876 ) ;
#26753=CIRCLE ( 'NONE', #11801, 9.084132297865673777 ) ;
#26755=CARTESIAN_POINT ( 'NONE',  ( 5.349779314757592275, 7.341751895053254096, -1.500000000000000888 ) ) ;
#26757=ORIENTED_EDGE ( 'NONE', *, *, #1735, .T. ) ;
#26764=DIRECTION ( 'NONE',  ( 0.000000000000000000, 1.000000000000000000, 1.132880637372608986E-16 ) ) ;
#26774=CYLINDRICAL_SURFACE ( 'NONE', #20018, 0.7500000000000006661 ) ;
#26779=ORIENTED_EDGE ( 'NONE', *, *, #22387, .F. ) ;
#26787=VECTOR ( 'NONE', #8940, 1000.000000000000000 ) ;
#26790=FACE_OUTER_BOUND ( 'NONE', #3509, .T. ) ;
#26802=CIRCLE ( 'NONE', #14326, 9.084132297865673777 ) ;
#26810=AXIS2_PLACEMENT_3D ( 'NONE', #20190, #5699, #3208 ) ;
#26817=VECTOR ( 'NONE', #2335, 1000.000000000000000 ) ;
#26831=CARTESIAN_POINT ( 'NONE',  ( 6.364020599487797192, -6.482337650448430466, 13.22130136205108819 ) ) ;
#26839=CARTESIAN_POINT ( 'NONE',  ( -6.543385983536389894, -6.301234758012572712, -1.500000000000002442 ) ) ;
#26840=EDGE_CURVE ( 'NONE', #13097, #18592, #30577, .T. ) ;
#26842=AXIS2_PLACEMENT_3D ( 'NONE', #12087, #21899, #21586 ) ;
#26846=AXIS2_PLACEMENT_3D ( 'NONE', #15149, #19996, #10793 ) ;
#26855=VERTEX_POINT ( 'NONE', #19654 ) ;
#26865=DIRECTION ( 'NONE',  ( 1.000000000000000000, 0.000000000000000000, 0.000000000000000000 ) ) ;
#26866=CIRCLE ( 'NONE', #27868, 9.084132297865673777 ) ;
#26879=ORIENTED_EDGE ( 'NONE', *, *, #18423, .T. ) ;
#26887=ORIENTED_EDGE ( 'NONE', *, *, #16781, .F. ) ;
#26897=DIRECTION ( 'NONE',  ( 0.000000000000000000, 1.000000000000000000, 1.193512090021232842E-16 ) ) ;
#26899=DIRECTION ( 'NONE',  ( 0.000000000000000000, 1.000000000000000000, 0.000000000000000000 ) ) ;
#26927=DIRECTION ( 'NONE',  ( 1.000000000000000000, 0.000000000000000000, 0.000000000000000000 ) ) ;
#26941=DIRECTION ( 'NONE',  ( -0.000000000000000000, 1.132880637372608986E-16, -1.000000000000000000 ) ) ;
#26947=EDGE_CURVE ( 'NONE', #29162, #23828, #25538, .T. ) ;
#26964=AXIS2_PLACEMENT_3D ( 'NONE', #27405, #29580, #13055 ) ;
#26990=DIRECTION ( 'NONE',  ( 0.000000000000000000, 1.000000000000000000, 0.000000000000000000 ) ) ;
#26993=DIRECTION ( 'NONE',  ( 0.000000000000000000, 1.000000000000000000, 0.000000000000000000 ) ) ;
#27006=DIRECTION ( 'NONE',  ( -0.000000000000000000, -0.000000000000000000, 1.000000000000000000 ) ) ;
#27022=DIRECTION ( 'NONE',  ( 1.000000000000000000, 0.000000000000000000, 0.000000000000000000 ) ) ;
#27035=CIRCLE ( 'NONE', #20541, 9.084132297865673777 ) ;
#27036=ORIENTED_EDGE ( 'NONE', *, *, #4607, .T. ) ;
#27042=DIRECTION ( 'NONE',  ( 0.000000000000000000, -1.132880637372608986E-16, 1.000000000000000000 ) ) ;
#27045=EDGE_CURVE ( 'NONE', #7648, #7334, #11591, .T. ) ;
#27047=CARTESIAN_POINT ( 'NONE',  ( 8.884323311075775109, 1.438332125858202692, 21.50000000000000000 ) ) ;
#27055=AXIS2_PLACEMENT_3D ( 'NONE', #9740, #6638, #16153 ) ;
#27086=DIRECTION ( 'NONE',  ( 0.000000000000000000, 0.000000000000000000, 1.000000000000000000 ) ) ;
#27087=CARTESIAN_POINT ( 'NONE',  ( -2.270234684139619485, 8.795879380940586856, -1.500000000000000666 ) ) ;
#27099=LINE ( 'NONE', #1209, #20865 ) ;
#27115=ORIENTED_EDGE ( 'NONE', *, *, #14003, .T. ) ;
#27125=DIRECTION ( 'NONE',  ( 0.000000000000000000, 0.000000000000000000, 1.000000000000000000 ) ) ;
#27135=DIRECTION ( 'NONE',  ( 1.000000000000000000, 0.000000000000000000, 0.000000000000000000 ) ) ;
#27140=AXIS2_PLACEMENT_3D ( 'NONE', #15388, #3548, #9141 ) ;
#27141=CARTESIAN_POINT ( 'NONE',  ( -7.749586724479453181, -2.959227181723774525, -3.621320343559650379 ) ) ;
#27162=CARTESIAN_POINT ( 'NONE',  ( 2.431858781452735485, 8.752572334588128555, 13.22130136205108997 ) ) ;
#27193=CARTESIAN_POINT ( 'NONE',  ( 9.062880100047298271, 0.6210184355499750453, 21.50000000000000000 ) ) ;
#27205=DIRECTION ( 'NONE',  ( 1.000000000000000000, 0.000000000000000000, 0.000000000000000000 ) ) ;
#27207=ORIENTED_EDGE ( 'NONE', *, *, #28306, .T. ) ;
#27208=CARTESIAN_POINT ( 'NONE',  ( 0.000000000000000000, -1.324687536737320328E-14, 29.43090101791767665 ) ) ;
#27233=CIRCLE ( 'NONE', #21242, 9.084132297865673777 ) ;
#27243=ORIENTED_EDGE ( 'NONE', *, *, #21022, .T. ) ;
#27266=CIRCLE ( 'NONE', #12329, 0.7500000000000006661 ) ;
#27278=ORIENTED_EDGE ( 'NONE', *, *, #2301, .T. ) ;
#27285=ORIENTED_EDGE ( 'NONE', *, *, #1560, .T. ) ;
#27287=EDGE_CURVE ( 'NONE', #14759, #1559, #6627, .T. ) ;
#27309=VERTEX_POINT ( 'NONE', #8406 ) ;
#27310=EDGE_CURVE ( 'NONE', #29057, #11684, #15234, .T. ) ;
#27315=DIRECTION ( 'NONE',  ( -0.000000000000000000, 1.132880637372608986E-16, -1.000000000000000000 ) ) ;
#27328=VERTEX_POINT ( 'NONE', #10731 ) ;
#27344=CARTESIAN_POINT ( 'NONE',  ( 2.516121109503181241, 8.728722367416590799, 13.22130136205108997 ) ) ;
#27368=VECTOR ( 'NONE', #20604, 1000.000000000000000 ) ;
#27392=FACE_OUTER_BOUND ( 'NONE', #5353, .T. ) ;
#27405=CARTESIAN_POINT ( 'NONE',  ( -2.959227181723746547, 8.499586724479465616, -3.621320343559650379 ) ) ;
#27406=CYLINDRICAL_SURFACE ( 'NONE', #3961, 0.7499999999999997780 ) ;
#27415=DIRECTION ( 'NONE',  ( 0.000000000000000000, 0.000000000000000000, 1.000000000000000000 ) ) ;
#27421=EDGE_LOOP ( 'NONE', ( #1426, #27036 ) ) ;
#27422=ORIENTED_EDGE ( 'NONE', *, *, #18316, .T. ) ;
#27435=CARTESIAN_POINT ( 'NONE',  ( -3.196529495465446402, -8.413215745754985875, -3.621320343559650379 ) ) ;
#27442=DIRECTION ( 'NONE',  ( 0.000000000000000000, 0.000000000000000000, 1.000000000000000000 ) ) ;
#27452=DIRECTION ( 'NONE',  ( 0.000000000000000000, -1.132880637372608986E-16, 1.000000000000000000 ) ) ;
#27453=CARTESIAN_POINT ( 'NONE',  ( 0.1262659238204208167, 8.999114229549594057, 21.50000000000000000 ) ) ;
#27455=ORIENTED_EDGE ( 'NONE', *, *, #2602, .F. ) ;
#27459=EDGE_LOOP ( 'NONE', ( #2196, #5624, #157, #10646 ) ) ;
#27468=CIRCLE ( 'NONE', #30439, 0.7500000000000006661 ) ;
#27471=DIRECTION ( 'NONE',  ( -0.000000000000000000, -0.000000000000000000, 1.000000000000000000 ) ) ;
#27482=ADVANCED_FACE ( 'NONE', ( #24222 ), #23183, .F. ) ;
#27491=VERTEX_POINT ( 'NONE', #15487 ) ;
#27497=VERTEX_POINT ( 'NONE', #12550 ) ;
#27499=LINE ( 'NONE', #17666, #4306 ) ;
#27506=CARTESIAN_POINT ( 'NONE',  ( 0.000000000000000000, 15.00000000000001421, 117.5000000000000000 ) ) ;
#27509=DIRECTION ( 'NONE',  ( 0.000000000000000000, 1.000000000000000000, 0.000000000000000000 ) ) ;
#27528=CARTESIAN_POINT ( 'NONE',  ( 0.000000000000000000, 10.00000000000000888, 117.5000000000000000 ) ) ;
#27529=VECTOR ( 'NONE', #11979, 1000.000000000000000 ) ;
#27540=CARTESIAN_POINT ( 'NONE',  ( -8.499586724479453181, -2.959227181723774525, -1.500000000000002220 ) ) ;
#27543=ORIENTED_EDGE ( 'NONE', *, *, #2031, .F. ) ;
#27545=AXIS2_PLACEMENT_3D ( 'NONE', #9418, #7064, #16573 ) ;
#27546=AXIS2_PLACEMENT_3D ( 'NONE', #2989, #5165, #24495 ) ;
#27562=DIRECTION ( 'NONE',  ( 1.000000000000000000, 0.000000000000000000, -0.000000000000000000 ) ) ;
#27565=FACE_OUTER_BOUND ( 'NONE', #19188, .T. ) ;
#27572=DIRECTION ( 'NONE',  ( -0.000000000000000000, -0.000000000000000000, 1.000000000000000000 ) ) ;
#27609=EDGE_CURVE ( 'NONE', #25828, #7918, #15595, .T. ) ;
#27611=CARTESIAN_POINT ( 'NONE',  ( 0.000000000000000000, -9.742773481404436396E-15, -1.500000000000001332 ) ) ;
#27613=DIRECTION ( 'NONE',  ( 0.000000000000000000, 1.000000000000000000, 0.000000000000000000 ) ) ;
#27641=ORIENTED_EDGE ( 'NONE', *, *, #22171, .F. ) ;
#27656=DIRECTION ( 'NONE',  ( 0.000000000000000000, -1.132880637372608986E-16, 1.000000000000000000 ) ) ;
#27675=ORIENTED_EDGE ( 'NONE', *, *, #7927, .T. ) ;
#27683=DIRECTION ( 'NONE',  ( 0.000000000000000000, 1.132880637372608986E-16, -1.000000000000000000 ) ) ;
#27693=VECTOR ( 'NONE', #19210, 1000.000000000000000 ) ;
#27717=AXIS2_PLACEMENT_3D ( 'NONE', #27935, #1584, #13734 ) ;
#27724=DIRECTION ( 'NONE',  ( -5.782411586589351722E-15, 1.000000000000000000, 0.000000000000000000 ) ) ;
#27726=ORIENTED_EDGE ( 'NONE', *, *, #13464, .F. ) ;
#27727=CARTESIAN_POINT ( 'NONE',  ( -8.134323311075783991, -1.438332125858144295, -3.621320343559650379 ) ) ;
#27741=FACE_OUTER_BOUND ( 'NONE', #20156, .T. ) ;
#27761=CARTESIAN_POINT ( 'NONE',  ( 0.8750451464062524165, 9.041888939645138734, 21.50000000000000000 ) ) ;
#27776=CIRCLE ( 'NONE', #20313, 0.7500000000000006661 ) ;
#27794=CARTESIAN_POINT ( 'NONE',  ( 3.914781618004695041, 8.197313248159959542, 21.50000000000000000 ) ) ;
#27799=DIRECTION ( 'NONE',  ( 1.000000000000000000, 0.000000000000000000, 0.000000000000000000 ) ) ;
#27811=VECTOR ( 'NONE', #4310, 1000.000000000000000 ) ;
#27815=AXIS2_PLACEMENT_3D ( 'NONE', #13917, #13315, #25768 ) ;
#27818=FACE_OUTER_BOUND ( 'NONE', #29678, .T. ) ;
#27827=DIRECTION ( 'NONE',  ( 1.000000000000000000, 0.000000000000000000, 0.000000000000000000 ) ) ;
#27843=EDGE_LOOP ( 'NONE', ( #29845, #3577, #15374, #24563 ) ) ;
#27859=CARTESIAN_POINT ( 'NONE',  ( 7.730328572437743517, -4.608906612435629491, 21.50000000000000000 ) ) ;
#27863=EDGE_CURVE ( 'NONE', #14718, #3254, #4243, .T. ) ;
#27868=AXIS2_PLACEMENT_3D ( 'NONE', #6180, #8214, #15532 ) ;
#27879=EDGE_CURVE ( 'NONE', #26463, #12314, #13919, .T. ) ;
#27881=EDGE_CURVE ( 'NONE', #2587, #7648, #27776, .T. ) ;
#27882=ORIENTED_EDGE ( 'NONE', *, *, #6309, .T. ) ;
#27900=CARTESIAN_POINT ( 'NONE',  ( 0.1262659238204208167, 8.999114229549594057, 21.50000000000000000 ) ) ;
#27918=CARTESIAN_POINT ( 'NONE',  ( 0.000000000000000000, 9.738409107444585544, 27.94260272410217638 ) ) ;
#27921=ORIENTED_EDGE ( 'NONE', *, *, #21757, .T. ) ;
#27922=ADVANCED_FACE ( 'NONE', ( #21688 ), #7521, .F. ) ;
#27933=ORIENTED_EDGE ( 'NONE', *, *, #10325, .T. ) ;
#27935=CARTESIAN_POINT ( 'NONE',  ( -5.687793815610304726, 6.974883619896852238, -1.500000000000000888 ) ) ;
#27939=VERTEX_POINT ( 'NONE', #19053 ) ;
#27954=ORIENTED_EDGE ( 'NONE', *, *, #8074, .F. ) ;
#27955=DIRECTION ( 'NONE',  ( 0.000000000000000000, 1.132880637372608986E-16, -1.000000000000000000 ) ) ;
#27958=CIRCLE ( 'NONE', #1624, 0.7500000000000006661 ) ;
#27959=UNCERTAINTY_MEASURE_WITH_UNIT (LENGTH_MEASURE( 1.000000000000000082E-05 ), #4005, 'distance_accuracy_value', 'NONE');
#27979=CARTESIAN_POINT ( 'NONE',  ( -5.278755796068720585, -7.392982946727063798, 13.22130136205108819 ) ) ;
#27982=EDGE_LOOP ( 'NONE', ( #473, #11456, #19352, #27675 ) ) ;
#27985=DIRECTION ( 'NONE',  ( 0.000000000000000000, 0.000000000000000000, 1.000000000000000000 ) ) ;
#27987=VECTOR ( 'NONE', #5500, 1000.000000000000000 ) ;
#27992=AXIS2_PLACEMENT_3D ( 'NONE', #14977, #12183, #24014 ) ;
#27998=CYLINDRICAL_SURFACE ( 'NONE', #23185, 0.7500000000000006661 ) ;
#28009=VERTEX_POINT ( 'NONE', #26070 ) ;
#28013=EDGE_LOOP ( 'NONE', ( #2514, #16811, #22563, #19228 ) ) ;
#28024=AXIS2_PLACEMENT_3D ( 'NONE', #14110, #9747, #88 ) ;
#28030=VERTEX_POINT ( 'NONE', #19200 ) ;
#28044=VERTEX_POINT ( 'NONE', #24815 ) ;
#28047=AXIS2_PLACEMENT_3D ( 'NONE', #28933, #12559, #22051 ) ;
#28050=CARTESIAN_POINT ( 'NONE',  ( 7.538175180318423152, 5.069257791428403159, 13.22130136205108819 ) ) ;
#28055=EDGE_CURVE ( 'NONE', #10205, #28599, #6353, .T. ) ;
#28058=CARTESIAN_POINT ( 'NONE',  ( 4.390207617113956573, -7.856594496258208160, -1.500000000000002665 ) ) ;
#28059=VERTEX_POINT ( 'NONE', #10623 ) ;
#28087=DIRECTION ( 'NONE',  ( 0.000000000000000000, 0.000000000000000000, 1.000000000000000000 ) ) ;
#28098=ADVANCED_FACE ( 'NONE', ( #22619 ), #13729, .F. ) ;
#28106=EDGE_LOOP ( 'NONE', ( #5045, #6383 ) ) ;
#28123=DIRECTION ( 'NONE',  ( 0.000000000000000000, 1.000000000000000000, 0.000000000000000000 ) ) ;
#28144=ORIENTED_EDGE ( 'NONE', *, *, #15805, .T. ) ;
#28148=CYLINDRICAL_SURFACE ( 'NONE', #30071, 0.7500000000000006661 ) ;
#28152=DIRECTION ( 'NONE',  ( 0.000000000000000000, 1.000000000000000000, 0.000000000000000000 ) ) ;
#28162=ORIENTED_EDGE ( 'NONE', *, *, #20033, .F. ) ;
#28190=FACE_OUTER_BOUND ( 'NONE', #27459, .T. ) ;
#28196=EDGE_CURVE ( 'NONE', #27328, #20523, #24775, .T. ) ;
#28199=VECTOR ( 'NONE', #11602, 1000.000000000000000 ) ;
#28204=DIRECTION ( 'NONE',  ( -0.000000000000000000, 1.132880637372608986E-16, -1.000000000000000000 ) ) ;
#28205=VERTEX_POINT ( 'NONE', #23843 ) ;
#28207=ORIENTED_EDGE ( 'NONE', *, *, #24240, .T. ) ;
#28215=EDGE_CURVE ( 'NONE', #21196, #9030, #23277, .T. ) ;
#28216=AXIS2_PLACEMENT_3D ( 'NONE', #10987, #20635, #30154 ) ;
#28224=CARTESIAN_POINT ( 'NONE',  ( 0.000000000000000000, -3.165563358393047634E-15, 27.94260272410217638 ) ) ;
#28233=DIRECTION ( 'NONE',  ( 0.000000000000000000, 0.000000000000000000, 1.000000000000000000 ) ) ;
#28241=CARTESIAN_POINT ( 'NONE',  ( 8.303920738747214259, 3.683253992019856149, 13.22130136205108819 ) ) ;
#28250=EDGE_CURVE ( 'NONE', #28714, #11382, #9503, .T. ) ;
#28264=CIRCLE ( 'NONE', #877, 0.7500000000000011102 ) ;
#28274=AXIS2_PLACEMENT_3D ( 'NONE', #12786, #5459, #928 ) ;
#28276=DIRECTION ( 'NONE',  ( 0.000000000000000000, 1.000000000000000000, 1.193512090021232842E-16 ) ) ;
#28278=ORIENTED_EDGE ( 'NONE', *, *, #1859, .T. ) ;
#28287=VECTOR ( 'NONE', #23316, 1000.000000000000000 ) ;
#28292=EDGE_CURVE ( 'NONE', #12174, #19662, #25809, .T. ) ;
#28297=CARTESIAN_POINT ( 'NONE',  ( 7.730328572437743517, -4.608906612435629491, 21.50000000000000000 ) ) ;
#28298=CARTESIAN_POINT ( 'NONE',  ( 6.482337650448408262, 6.364020599487815844, -1.500000000000001110 ) ) ;
#28301=VERTEX_POINT ( 'NONE', #30303 ) ;
#28305=AXIS2_PLACEMENT_3D ( 'NONE', #23365, #4793, #23509 ) ;
#28306=EDGE_CURVE ( 'NONE', #29624, #25948, #26802, .T. ) ;
#28318=AXIS2_PLACEMENT_3D ( 'NONE', #10344, #22491, #15320 ) ;
#28327=ORIENTED_EDGE ( 'NONE', *, *, #19894, .T. ) ;
#28337=VERTEX_POINT ( 'NONE', #4105 ) ;
#28344=CARTESIAN_POINT ( 'NONE',  ( -8.728722367416567707, 2.516121109503271835, 21.50000000000000000 ) ) ;
#28345=CARTESIAN_POINT ( 'NONE',  ( -8.999114229549592281, 0.1262659238205133538, 21.50000000000000000 ) ) ;
#28353=DIRECTION ( 'NONE',  ( 1.000000000000000000, 0.000000000000000000, 0.000000000000000000 ) ) ;
#28360=DIRECTION ( 'NONE',  ( 1.000000000000000000, 0.000000000000000000, 0.000000000000000000 ) ) ;
#28364=CARTESIAN_POINT ( 'NONE',  ( -2.446529495465445958, -8.413215745754985875, -1.500000000000002665 ) ) ;
#28375=LINE ( 'NONE', #4966, #11992 ) ;
#28378=ORIENTED_EDGE ( 'NONE', *, *, #25764, .T. ) ;
#28379=CIRCLE ( 'NONE', #23398, 9.084132297865673777 ) ;
#28392=CARTESIAN_POINT ( 'NONE',  ( 4.608906612435600181, 7.730328572437758616, 21.50000000000000000 ) ) ;
#28400=CIRCLE ( 'NONE', #13991, 7.500000000000008882 ) ;
#28408=CARTESIAN_POINT ( 'NONE',  ( -6.364020599487749230, 6.482337650448472210, 21.50000000000000000 ) ) ;
#28412=EDGE_CURVE ( 'NONE', #19937, #11840, #6901, .T. ) ;
#28419=CIRCLE ( 'NONE', #8015, 9.084132297865673777 ) ;
#28430=EDGE_CURVE ( 'NONE', #23872, #10205, #11133, .T. ) ;
#28452=ADVANCED_FACE ( 'NONE', ( #4367 ), #1436, .F. ) ;
#28474=ORIENTED_EDGE ( 'NONE', *, *, #5920, .F. ) ;
#28478=ADVANCED_FACE ( 'NONE', ( #30707 ), #14494, .F. ) ;
#28490=DIRECTION ( 'NONE',  ( 1.000000000000000000, 0.000000000000000000, 0.000000000000000000 ) ) ;
#28496=CYLINDRICAL_SURFACE ( 'NONE', #16517, 15.00000000000003375 ) ;
#28505=DIRECTION ( 'NONE',  ( 0.000000000000000000, -1.132880637372608986E-16, 1.000000000000000000 ) ) ;
#28510=ORIENTED_EDGE ( 'NONE', *, *, #17391, .T. ) ;
#28514=DIRECTION ( 'NONE',  ( 0.000000000000000000, 0.000000000000000000, 1.000000000000000000 ) ) ;
#28515=EDGE_LOOP ( 'NONE', ( #25893, #7352, #19503, #19347 ) ) ;
#28516=ADVANCED_FACE ( 'NONE', ( #6865 ), #6258, .F. ) ;
#28517=PLANE ( 'NONE',  #5203 ) ;
#28521=AXIS2_PLACEMENT_3D ( 'NONE', #19298, #16802, #18998 ) ;
#28525=ORIENTED_EDGE ( 'NONE', *, *, #19110, .T. ) ;
#28527=ORIENTED_EDGE ( 'NONE', *, *, #17061, .F. ) ;
#28534=CARTESIAN_POINT ( 'NONE',  ( -7.538175180318458679, -5.069257791428355198, 13.22130136205108819 ) ) ;
#28537=AXIS2_PLACEMENT_3D ( 'NONE', #15499, #20638, #27205 ) ;
#28551=DIRECTION ( 'NONE',  ( -0.000000000000000000, 1.132880637372608986E-16, -1.000000000000000000 ) ) ;
#28557=CARTESIAN_POINT ( 'NONE',  ( -4.937793815610304726, 6.974883619896852238, -1.500000000000000888 ) ) ;
#28562=UNCERTAINTY_MEASURE_WITH_UNIT (LENGTH_MEASURE( 1.000000000000000082E-05 ), #18067, 'distance_accuracy_value', 'NONE');
#28571=VERTEX_POINT ( 'NONE', #8751 ) ;
#28575=DIRECTION ( 'NONE',  ( -0.000000000000000000, 1.132880637372608986E-16, -1.000000000000000000 ) ) ;
#28582=CIRCLE ( 'NONE', #7162, 9.084132297865673777 ) ;
#28592=FACE_OUTER_BOUND ( 'NONE', #12006, .T. ) ;
#28599=VERTEX_POINT ( 'NONE', #2649 ) ;
#28606=DIRECTION ( 'NONE',  ( 0.000000000000000000, 0.000000000000000000, 1.000000000000000000 ) ) ;
#28607=DIRECTION ( 'NONE',  ( 0.000000000000000000, 1.132880637372608986E-16, -1.000000000000000000 ) ) ;
#28608=CARTESIAN_POINT ( 'NONE',  ( -5.278755796068720585, -7.392982946727063798, 21.50000000000000000 ) ) ;
#28614=ORIENTED_EDGE ( 'NONE', *, *, #25767, .F. ) ;
#28630=ADVANCED_FACE ( 'NONE', ( #12016 ), #7338, .F. ) ;
#28644=ADVANCED_FACE ( 'NONE', ( #11802 ), #20692, .F. ) ;
#28650=DIRECTION ( 'NONE',  ( -0.000000000000000000, -0.000000000000000000, 1.000000000000000000 ) ) ;
#28653=FACE_OUTER_BOUND ( 'NONE', #6066, .T. ) ;
#28657=EDGE_LOOP ( 'NONE', ( #23133, #23478, #726, #21819 ) ) ;
#28659=ADVANCED_FACE ( 'NONE', ( #16177 ), #4168, .F. ) ;
#28661=CYLINDRICAL_SURFACE ( 'NONE', #28521, 0.7500000000000006661 ) ;
#28662=ORIENTED_EDGE ( 'NONE', *, *, #21943, .T. ) ;
#28664=ORIENTED_EDGE ( 'NONE', *, *, #3506, .F. ) ;
#28667=ADVANCED_FACE ( 'NONE', ( #8863 ), #4632, .F. ) ;
#28678=ORIENTED_EDGE ( 'NONE', *, *, #1232, .T. ) ;
#28683=EDGE_CURVE ( 'NONE', #19990, #6231, #16832, .T. ) ;
#28696=FACE_OUTER_BOUND ( 'NONE', #14432, .T. ) ;
#28710=DIRECTION ( 'NONE',  ( 0.000000000000000000, 0.000000000000000000, 1.000000000000000000 ) ) ;
#28712=CIRCLE ( 'NONE', #2294, 0.7499999999999997780 ) ;
#28713=DIRECTION ( 'NONE',  ( 1.000000000000000000, 0.000000000000000000, 0.000000000000000000 ) ) ;
#28714=VERTEX_POINT ( 'NONE', #13697 ) ;
#28716=AXIS2_PLACEMENT_3D ( 'NONE', #18462, #27656, #27509 ) ;
#28738=LINE ( 'NONE', #5027, #20197 ) ;
#28742=EDGE_LOOP ( 'NONE', ( #22953, #29740, #23513, #15600 ) ) ;
#28755=VECTOR ( 'NONE', #6544, 1000.000000000000000 ) ;
#28756=EDGE_LOOP ( 'NONE', ( #8280, #5521, #12539, #21758 ) ) ;
#28776=AXIS2_PLACEMENT_3D ( 'NONE', #7268, #26617, #16780 ) ;
#28791=AXIS2_PLACEMENT_3D ( 'NONE', #16071, #27471, #20445 ) ;
#28798=DIRECTION ( 'NONE',  ( 1.000000000000000000, 0.000000000000000000, -0.000000000000000000 ) ) ;
#28800=VECTOR ( 'NONE', #29679, 1000.000000000000000 ) ;
#28812=DIRECTION ( 'NONE',  ( -0.000000000000000000, -0.000000000000000000, 1.000000000000000000 ) ) ;
#28816=AXIS2_PLACEMENT_3D ( 'NONE', #3643, #8497, #677 ) ;
#28820=AXIS2_PLACEMENT_3D ( 'NONE', #8066, #10552, #1196 ) ;
#28821=ORIENTED_EDGE ( 'NONE', *, *, #27863, .T. ) ;
#28835=ADVANCED_FACE ( 'NONE', ( #2760 ), #19591, .F. ) ;
#28839=EDGE_CURVE ( 'NONE', #28714, #11459, #6899, .T. ) ;
#28850=DIRECTION ( 'NONE',  ( 1.000000000000000000, 0.000000000000000000, -0.000000000000000000 ) ) ;
#28851=EDGE_LOOP ( 'NONE', ( #5108, #10376 ) ) ;
#28855=DIRECTION ( 'NONE',  ( -0.000000000000000000, -0.000000000000000000, 1.000000000000000000 ) ) ;
#28870=CARTESIAN_POINT ( 'NONE',  ( 0.000000000000000000, 9.084132297865670225, 27.94260272410217638 ) ) ;
#28871=CIRCLE ( 'NONE', #12423, 0.7500000000000006661 ) ;
#28873=DIRECTION ( 'NONE',  ( 0.000000000000000000, 0.000000000000000000, 1.000000000000000000 ) ) ;
#28880=CYLINDRICAL_SURFACE ( 'NONE', #27992, 0.7500000000000002220 ) ;
#28891=AXIS2_PLACEMENT_3D ( 'NONE', #9109, #27985, #23587 ) ;
#28897=DIRECTION ( 'NONE',  ( -0.000000000000000000, -0.000000000000000000, 1.000000000000000000 ) ) ;
#28898=CIRCLE ( 'NONE', #7479, 9.084132297865673777 ) ;
#28903=CARTESIAN_POINT ( 'NONE',  ( 0.000000000000000000, 1.699320956058915452E-16, -1.500000000000001776 ) ) ;
#28904=VERTEX_POINT ( 'NONE', #29723 ) ;
#28927=CARTESIAN_POINT ( 'NONE',  ( -8.840471615930058036, 1.687027447297517080, -3.621320343559650379 ) ) ;
#28932=AXIS2_PLACEMENT_3D ( 'NONE', #28058, #30094, #30403 ) ;
#28933=CARTESIAN_POINT ( 'NONE',  ( -6.974883619896829146, -5.687793815610328707, -3.621320343559650379 ) ) ;
#28938=VECTOR ( 'NONE', #22340, 1000.000000000000000 ) ;
#28944=CARTESIAN_POINT ( 'NONE',  ( 5.881244434206234217, 6.812559277181991391, 21.50000000000000000 ) ) ;
#28969=EDGE_LOOP ( 'NONE', ( #4707, #10645, #11223 ) ) ;
#28987=EDGE_CURVE ( 'NONE', #25828, #7554, #18493, .T. ) ;
#29021=CARTESIAN_POINT ( 'NONE',  ( -8.884323311075783991, -1.438332125858144295, -1.500000000000001776 ) ) ;
#29025=AXIS2_PLACEMENT_3D ( 'NONE', #21342, #25584, #16369 ) ;
#29027=AXIS2_PLACEMENT_3D ( 'NONE', #4496, #23811, #5106 ) ;
#29038=ORIENTED_EDGE ( 'NONE', *, *, #1521, .T. ) ;
#29050=LINE ( 'NONE', #7693, #11046 ) ;
#29057=VERTEX_POINT ( 'NONE', #6772 ) ;
#29061=EDGE_LOOP ( 'NONE', ( #20568, #8517 ) ) ;
#29071=CARTESIAN_POINT ( 'NONE',  ( 8.728722367416583694, -2.516121109503213216, 21.50000000000000000 ) ) ;
#29076=ADVANCED_FACE ( 'NONE', ( #4590 ), #20512, .T. ) ;
#29091=VERTEX_POINT ( 'NONE', #17211 ) ;
#29107=LINE ( 'NONE', #710, #15794 ) ;
#29117=DIRECTION ( 'NONE',  ( 1.000000000000000000, 0.000000000000000000, 0.000000000000000000 ) ) ;
#29128=ORIENTED_EDGE ( 'NONE', *, *, #13613, .F. ) ;
#29145=DIRECTION ( 'NONE',  ( -3.469446951953611033E-15, 1.000000000000000000, 0.000000000000000000 ) ) ;
#29154=VERTEX_POINT ( 'NONE', #29071 ) ;
#29157=CARTESIAN_POINT ( 'NONE',  ( -8.840471615930058036, 1.687027447297517080, 21.50000000000000000 ) ) ;
#29162=VERTEX_POINT ( 'NONE', #9437 ) ;
#29173=ORIENTED_EDGE ( 'NONE', *, *, #15315, .F. ) ;
#29202=ORIENTED_EDGE ( 'NONE', *, *, #2678, .T. ) ;
#29210=ORIENTED_EDGE ( 'NONE', *, *, #20067, .F. ) ;
#29213=CIRCLE ( 'NONE', #9283, 0.7500000000000004441 ) ;
#29216=AXIS2_PLACEMENT_3D ( 'NONE', #12832, #5963, #10791 ) ;
#29226=CARTESIAN_POINT ( 'NONE',  ( 0.000000000000000000, 1.699320956058915452E-16, -1.500000000000001776 ) ) ;
#29231=VECTOR ( 'NONE', #222, 1000.000000000000000 ) ;
#29272=DIRECTION ( 'NONE',  ( -8.962737959213495958E-15, 1.000000000000000000, 0.000000000000000000 ) ) ;
#29277=ORIENTED_EDGE ( 'NONE', *, *, #1549, .T. ) ;
#29286=AXIS2_PLACEMENT_3D ( 'NONE', #1593, #28087, #11244 ) ;
#29300=DIRECTION ( 'NONE',  ( 0.000000000000000000, 1.132880637372608986E-16, -1.000000000000000000 ) ) ;
#29312=FACE_OUTER_BOUND ( 'NONE', #5192, .T. ) ;
#29324=CARTESIAN_POINT ( 'NONE',  ( 5.881244434206234217, 6.812559277181991391, -1.500000000000000888 ) ) ;
#29341=ORIENTED_EDGE ( 'NONE', *, *, #17756, .F. ) ;
#29358=VERTEX_POINT ( 'NONE', #3181 ) ;
#29369=DIRECTION ( 'NONE',  ( 0.000000000000000000, 0.000000000000000000, 1.000000000000000000 ) ) ;
#29382=EDGE_CURVE ( 'NONE', #11001, #20003, #11873, .T. ) ;
#29384=ORIENTED_EDGE ( 'NONE', *, *, #24439, .T. ) ;
#29389=FACE_OUTER_BOUND ( 'NONE', #352, .T. ) ;
#29400=DIRECTION ( 'NONE',  ( -0.000000000000000000, 1.132880637372608986E-16, -1.000000000000000000 ) ) ;
#29402=EDGE_CURVE ( 'NONE', #20812, #3530, #5904, .T. ) ;
#29412=ORIENTED_EDGE ( 'NONE', *, *, #16087, .T. ) ;
#29417=CIRCLE ( 'NONE', #2512, 12.18947652193948272 ) ;
#29427=CARTESIAN_POINT ( 'NONE',  ( -7.663215745754974328, 3.196529495465474380, 21.50000000000000000 ) ) ;
#29438=VERTEX_POINT ( 'NONE', #19366 ) ;
#29443=EDGE_CURVE ( 'NONE', #23362, #5775, #26340, .T. ) ;
#29449=AXIS2_PLACEMENT_3D ( 'NONE', #12545, #22036, #10041 ) ;
#29460=( NAMED_UNIT ( * ) SI_UNIT ( $, .STERADIAN. ) SOLID_ANGLE_UNIT ( ) );
#29471=EDGE_CURVE ( 'NONE', #11152, #21957, #11726, .T. ) ;
#29486=CARTESIAN_POINT ( 'NONE',  ( -8.999114229549592281, 0.1262659238205133538, -1.500000000000001776 ) ) ;
#29493=FACE_OUTER_BOUND ( 'NONE', #9490, .T. ) ;
#29504=CIRCLE ( 'NONE', #16051, 0.7500000000000006661 ) ;
#29509=ORIENTED_EDGE ( 'NONE', *, *, #2301, .F. ) ;
#29510=EDGE_CURVE ( 'NONE', #29358, #1662, #10308, .T. ) ;
#29514=CYLINDRICAL_SURFACE ( 'NONE', #1813, 0.7500000000000003331 ) ;
#29523=ORIENTED_EDGE ( 'NONE', *, *, #23115, .F. ) ;
#29540=DIRECTION ( 'NONE',  ( 0.000000000000000000, -1.132880637372608986E-16, 1.000000000000000000 ) ) ;
#29548=CYLINDRICAL_SURFACE ( 'NONE', #2639, 0.7499999999999997780 ) ;
#29560=FACE_BOUND ( 'NONE', #17550, .T. ) ;
#29578=DIRECTION ( 'NONE',  ( 0.000000000000000000, -1.132880637372608986E-16, 1.000000000000000000 ) ) ;
#29580=DIRECTION ( 'NONE',  ( -0.000000000000000000, -0.000000000000000000, 1.000000000000000000 ) ) ;
#29581=PLANE ( 'NONE',  #20877 ) ;
#29586=ORIENTED_EDGE ( 'NONE', *, *, #1601, .F. ) ;
#29587=EDGE_LOOP ( 'NONE', ( #1700, #18544, #17395, #22930 ) ) ;
#29602=ORIENTED_EDGE ( 'NONE', *, *, #21615, .T. ) ;
#29606=ORIENTED_EDGE ( 'NONE', *, *, #19089, .T. ) ;
#29611=CARTESIAN_POINT ( 'NONE',  ( 8.795879380940563763, 2.270234684139707859, 13.22130136205108819 ) ) ;
#29614=EDGE_CURVE ( 'NONE', #4424, #191, #22841, .T. ) ;
#29617=DIRECTION ( 'NONE',  ( 0.000000000000000000, 1.132880637372608986E-16, -1.000000000000000000 ) ) ;
#29624=VERTEX_POINT ( 'NONE', #10199 ) ;
#29629=ORIENTED_EDGE ( 'NONE', *, *, #20788, .F. ) ;
#29678=EDGE_LOOP ( 'NONE', ( #22922, #25847, #18966, #14557 ) ) ;
#29679=DIRECTION ( 'NONE',  ( 0.000000000000000000, -1.132880637372608986E-16, 1.000000000000000000 ) ) ;
#29698=EDGE_LOOP ( 'NONE', ( #25222, #11131, #28474 ) ) ;
#29709=VECTOR ( 'NONE', #25292, 1000.000000000000000 ) ;
#29710=ORIENTED_EDGE ( 'NONE', *, *, #789, .T. ) ;
#29712=FACE_OUTER_BOUND ( 'NONE', #28515, .T. ) ;
#29723=CARTESIAN_POINT ( 'NONE',  ( -2.446529495465445958, -8.413215745754985875, 21.50000000000000000 ) ) ;
#29732=AXIS2_PLACEMENT_3D ( 'NONE', #24712, #8194, #26764 ) ;
#29736=DIRECTION ( 'NONE',  ( 0.000000000000000000, 0.000000000000000000, 1.000000000000000000 ) ) ;
#29737=LINE ( 'NONE', #17723, #21100 ) ;
#29740=ORIENTED_EDGE ( 'NONE', *, *, #12865, .T. ) ;
#29743=CARTESIAN_POINT ( 'NONE',  ( 1.224646799147357201E-15, -10.00000000000003375, -87.50000000000000000 ) ) ;
#29745=ORIENTED_EDGE ( 'NONE', *, *, #11878, .T. ) ;
#29757=EDGE_LOOP ( 'NONE', ( #8880, #28821, #28510, #24517, #21304, #18653, #20650, #21473, #11699, #6343, #22921, #7273, #17430, #7472, #28378, #12070, #15591, #21004, #23978, #1261, #5684, #27278, #25595, #17882, #19578, #8007, #11220, #5809, #14573, #25008, #5726, #22126, #6237, #19108, #26879, #26215, #19229, #22456, #29277, #18643, #1703, #1021, #16433, #10518, #28162, #10281, #29384, #22639, #4899, #21222, #1438, #25374, #18981, #20416, #20749, #24383, #26058, #12907, #12493, #7823, #20207, #3754, #6551, #8316, #14212, #24739, #4751, #8485, #27543, #13690, #13081, #21783, #22052, #20925, #1065, #21072 ) ) ;
#29761=AXIS2_PLACEMENT_3D ( 'NONE', #25908, #27955, #16541 ) ;
#29769=CIRCLE ( 'NONE', #28274, 0.7500000000000006661 ) ;
#29772=EDGE_CURVE ( 'NONE', #8229, #30243, #7720, .T. ) ;
#29779=AXIS2_PLACEMENT_3D ( 'NONE', #10309, #7821, #22463 ) ;
#29782=CIRCLE ( 'NONE', #24778, 12.50000000000000000 ) ;
#29784=ORIENTED_EDGE ( 'NONE', *, *, #2360, .F. ) ;
#29791=LINE ( 'NONE', #8432, #17653 ) ;
#29796=ADVANCED_FACE ( 'NONE', ( #7239 ), #2726, .F. ) ;
#29818=DIRECTION ( 'NONE',  ( -0.000000000000000000, -0.000000000000000000, 1.000000000000000000 ) ) ;
#29845=ORIENTED_EDGE ( 'NONE', *, *, #9043, .F. ) ;
#29854=DIRECTION ( 'NONE',  ( 1.000000000000000000, 0.000000000000000000, 0.000000000000000000 ) ) ;
#29856=AXIS2_PLACEMENT_3D ( 'NONE', #9910, #24247, #12416 ) ;
#29867=EDGE_CURVE ( 'NONE', #21841, #27491, #22278, .T. ) ;
#29870=FACE_OUTER_BOUND ( 'NONE', #25690, .T. ) ;
#29882=CIRCLE ( 'NONE', #28891, 9.084132297865673777 ) ;
#29898=CYLINDRICAL_SURFACE ( 'NONE', #14409, 0.7500000000000004441 ) ;
#29905=ORIENTED_EDGE ( 'NONE', *, *, #21348, .T. ) ;
#29906=CARTESIAN_POINT ( 'NONE',  ( 4.390207617113956573, -7.856594496258208160, 21.50000000000000000 ) ) ;
#29909=ORIENTED_EDGE ( 'NONE', *, *, #24663, .T. ) ;
#29917=DIRECTION ( 'NONE',  ( 0.000000000000000000, 0.000000000000000000, 1.000000000000000000 ) ) ;
#29924=EDGE_LOOP ( 'NONE', ( #29173, #29586, #13617, #2148 ) ) ;
#29930=EDGE_CURVE ( 'NONE', #11382, #14759, #12837, .T. ) ;
#29939=CARTESIAN_POINT ( 'NONE',  ( -2.185336383880142730, 8.817355867515834333, 21.50000000000000000 ) ) ;
#29949=DIRECTION ( 'NONE',  ( 0.000000000000000000, 0.000000000000000000, 1.000000000000000000 ) ) ;
#29951=FACE_BOUND ( 'NONE', #7222, .T. ) ;
#29954=CARTESIAN_POINT ( 'NONE',  ( 0.1262659238204208167, 8.999114229549594057, -1.500000000000000888 ) ) ;
#29967=CARTESIAN_POINT ( 'NONE',  ( 0.000000000000000000, -8.043452525345523162E-15, -16.50000000000000000 ) ) ;
#29976=AXIS2_PLACEMENT_3D ( 'NONE', #21345, #16371, #23384 ) ;
#30006=CARTESIAN_POINT ( 'NONE',  ( 0.000000000000000000, 1.699320956058915452E-16, -1.500000000000001776 ) ) ;
#30020=CARTESIAN_POINT ( 'NONE',  ( 0.000000000000000000, 1.699320956058915452E-16, -1.500000000000001776 ) ) ;
#30039=CARTESIAN_POINT ( 'NONE',  ( -2.959227181723746547, 8.499586724479465616, 21.50000000000000000 ) ) ;
#30040=DIRECTION ( 'NONE',  ( -0.000000000000000000, 1.132880637372608986E-16, -1.000000000000000000 ) ) ;
#30043=CARTESIAN_POINT ( 'NONE',  ( 8.413215745754998309, -3.196529495465417980, 21.50000000000000000 ) ) ;
#30049=ORIENTED_EDGE ( 'NONE', *, *, #7497, .T. ) ;
#30054=ORIENTED_EDGE ( 'NONE', *, *, #11645, .F. ) ;
#30065=ADVANCED_FACE ( 'NONE', ( #14904 ), #5398, .F. ) ;
#30071=AXIS2_PLACEMENT_3D ( 'NONE', #27435, #3726, #25081 ) ;
#30079=CIRCLE ( 'NONE', #28024, 0.7500000000000004441 ) ;
#30088=CARTESIAN_POINT ( 'NONE',  ( -0.8750451464063154772, -9.041888939645135181, -1.500000000000002887 ) ) ;
#30091=ORIENTED_EDGE ( 'NONE', *, *, #20782, .T. ) ;
#30093=PLANE ( 'NONE',  #10775 ) ;
#30094=DIRECTION ( 'NONE',  ( 0.000000000000000000, -1.132880637372608986E-16, 1.000000000000000000 ) ) ;
#30095=ORIENTED_EDGE ( 'NONE', *, *, #16997, .F. ) ;
#30096=DIRECTION ( 'NONE',  ( 0.000000000000000000, 0.000000000000000000, 1.000000000000000000 ) ) ;
#30104=DIRECTION ( 'NONE',  ( 0.000000000000000000, 1.000000000000000000, 0.000000000000000000 ) ) ;
#30112=DIRECTION ( 'NONE',  ( 0.000000000000000000, 1.000000000000000000, 0.000000000000000000 ) ) ;
#30117=ORIENTED_EDGE ( 'NONE', *, *, #21033, .F. ) ;
#30121=CARTESIAN_POINT ( 'NONE',  ( -6.543385983536390782, -6.301234758012574488, 13.22130136205108819 ) ) ;
#30136=ORIENTED_EDGE ( 'NONE', *, *, #16120, .T. ) ;
#30140=CARTESIAN_POINT ( 'NONE',  ( 0.000000000000000000, -8.043452525345523162E-15, -16.50000000000000000 ) ) ;
#30151=CARTESIAN_POINT ( 'NONE',  ( 7.538175180318423152, 5.069257791428403159, -1.500000000000001110 ) ) ;
#30154=DIRECTION ( 'NONE',  ( 1.000000000000000000, 0.000000000000000000, 0.000000000000000000 ) ) ;
#30157=ORIENTED_EDGE ( 'NONE', *, *, #24828, .T. ) ;
#30159=AXIS2_PLACEMENT_3D ( 'NONE', #4535, #23405, #23698 ) ;
#30173=ADVANCED_FACE ( 'NONE', ( #29712 ), #8523, .F. ) ;
#30183=DIRECTION ( 'NONE',  ( -0.000000000000000000, -0.000000000000000000, 1.000000000000000000 ) ) ;
#30185=CARTESIAN_POINT ( 'NONE',  ( -0.6883321258581104329, 8.884323311075791096, 21.50000000000000000 ) ) ;
#30196=DIRECTION ( 'NONE',  ( 0.000000000000000000, 1.000000000000000000, 1.193512090021232842E-16 ) ) ;
#30199=CARTESIAN_POINT ( 'NONE',  ( -1.438332125858111432, 8.884323311075791096, -1.500000000000000888 ) ) ;
#30217=EDGE_LOOP ( 'NONE', ( #29210, #3426, #29341 ) ) ;
#30224=AXIS2_PLACEMENT_3D ( 'NONE', #2522, #11722, #167 ) ;
#30240=VECTOR ( 'NONE', #4866, 1000.000000000000000 ) ;
#30243=VERTEX_POINT ( 'NONE', #17700 ) ;
#30252=AXIS2_PLACEMENT_3D ( 'NONE', #246, #16168, #25845 ) ;
#30255=VECTOR ( 'NONE', #21535, 1000.000000000000000 ) ;
#30256=VERTEX_POINT ( 'NONE', #20186 ) ;
#30276=FACE_OUTER_BOUND ( 'NONE', #18685, .T. ) ;
#30279=VERTEX_POINT ( 'NONE', #6160 ) ;
#30288=DIRECTION ( 'NONE',  ( -1.156482317317873105E-15, 1.000000000000000000, 0.000000000000000000 ) ) ;
#30291=ORIENTED_EDGE ( 'NONE', *, *, #25987, .F. ) ;
#30303=CARTESIAN_POINT ( 'NONE',  ( 8.197313248159948884, -3.914781618004724795, 21.50000000000000000 ) ) ;
#30310=AXIS2_PLACEMENT_3D ( 'NONE', #23297, #1940, #2984 ) ;
#30374=VERTEX_POINT ( 'NONE', #650 ) ;
#30384=DIRECTION ( 'NONE',  ( 0.000000000000000000, -1.132880637372608986E-16, 1.000000000000000000 ) ) ;
#30401=CARTESIAN_POINT ( 'NONE',  ( 0.000000000000000000, 1.699320956058915452E-16, -1.500000000000001776 ) ) ;
#30403=DIRECTION ( 'NONE',  ( 0.000000000000000000, 1.000000000000000000, 0.000000000000000000 ) ) ;
#30419=CIRCLE ( 'NONE', #23933, 9.084132297865673777 ) ;
#30428=CARTESIAN_POINT ( 'NONE',  ( 0.000000000000000000, -9.742773481404436396E-15, -1.500000000000001332 ) ) ;
#30431=ORIENTED_EDGE ( 'NONE', *, *, #27879, .T. ) ;
#30439=AXIS2_PLACEMENT_3D ( 'NONE', #20538, #29917, #17912 ) ;
#30440=CARTESIAN_POINT ( 'NONE',  ( -7.730328572437709767, 4.608906612435681005, -3.621320343559650379 ) ) ;
#30444=FACE_OUTER_BOUND ( 'NONE', #13878, .T. ) ;
#30456=CARTESIAN_POINT ( 'NONE',  ( 2.185336383880204014, -8.817355867515821899, 13.22130136205108641 ) ) ;
#30463=CARTESIAN_POINT ( 'NONE',  ( -3.196529495465446402, -8.413215745754985875, 21.50000000000000000 ) ) ;
#30468=DIRECTION ( 'NONE',  ( -0.000000000000000000, -0.000000000000000000, 1.000000000000000000 ) ) ;
#30487=DIRECTION ( 'NONE',  ( 0.000000000000000000, 0.000000000000000000, 1.000000000000000000 ) ) ;
#30493=FACE_OUTER_BOUND ( 'NONE', #29924, .T. ) ;
#30508=AXIS2_PLACEMENT_3D ( 'NONE', #16708, #7041, #2671 ) ;
#30510=EDGE_CURVE ( 'NONE', #6357, #386, #6713, .T. ) ;
#30514=EDGE_LOOP ( 'NONE', ( #4986, #1566, #13431, #24874 ) ) ;
#30528=DIRECTION ( 'NONE',  ( 0.000000000000000000, 1.000000000000000000, 0.000000000000000000 ) ) ;
#30529=EDGE_CURVE ( 'NONE', #5002, #24171, #23541, .T. ) ;
#30543=DIRECTION ( 'NONE',  ( 0.000000000000000000, 1.132880637372608986E-16, -1.000000000000000000 ) ) ;
#30544=EDGE_LOOP ( 'NONE', ( #11184, #12062 ) ) ;
#30577=CIRCLE ( 'NONE', #27546, 0.7500000000000004441 ) ;
#30582=ORIENTED_EDGE ( 'NONE', *, *, #16791, .F. ) ;
#30590=DIRECTION ( 'NONE',  ( -0.000000000000000000, 1.132880637372608986E-16, -1.000000000000000000 ) ) ;
#30639=ORIENTED_EDGE ( 'NONE', *, *, #19013, .F. ) ;
#30643=ORIENTED_EDGE ( 'NONE', *, *, #17740, .T. ) ;
#30655=CARTESIAN_POINT ( 'NONE',  ( 0.000000000000000000, -2.435693370351110282E-15, 21.50000000000000355 ) ) ;
#30658=ORIENTED_EDGE ( 'NONE', *, *, #14265, .T. ) ;
#30661=FACE_OUTER_BOUND ( 'NONE', #18865, .T. ) ;
#30669=CYLINDRICAL_SURFACE ( 'NONE', #16877, 0.7500000000000006661 ) ;
#30676=AXIS2_PLACEMENT_3D ( 'NONE', #19026, #30706, #16376 ) ;
#30682=ADVANCED_FACE ( 'NONE', ( #24322 ), #19959, .F. ) ;
#30687=CARTESIAN_POINT ( 'NONE',  ( -7.538175180318456903, -5.069257791428354309, -1.500000000000002442 ) ) ;
#30688=AXIS2_PLACEMENT_3D ( 'NONE', #24309, #12476, #21966 ) ;
#30706=DIRECTION ( 'NONE',  ( 0.000000000000000000, 0.000000000000000000, 1.000000000000000000 ) ) ;
#30707=FACE_OUTER_BOUND ( 'NONE', #513, .T. ) ;
#30709=PLANE ( 'NONE',  #25761 ) ;
#30720=DIRECTION ( 'NONE',  ( -0.000000000000000000, 1.132880637372608986E-16, -1.000000000000000000 ) ) ;
#30724=CYLINDRICAL_SURFACE ( 'NONE', #10937, 0.7500000000000006661 ) ;
#30727=AXIS2_PLACEMENT_3D ( 'NONE', #4526, #23851, #14036 ) ;
#30730=CARTESIAN_POINT ( 'NONE',  ( -5.881244434206279514, -6.812559277181949646, 21.50000000000000000 ) ) ;
#30734=ORIENTED_EDGE ( 'NONE', *, *, #9001, .T. ) ;
#30735=EDGE_CURVE ( 'NONE', #6045, #23454, #15853, .T. ) ;
#30748=CARTESIAN_POINT ( 'NONE',  ( 0.000000000000000000, 9.084132297865666672, 65.52304386563415051 ) ) ;
#30749=CARTESIAN_POINT ( 'NONE',  ( -0.1262659238204836554, -8.999114229549588728, -1.500000000000002665 ) ) ;
#30754=AXIS2_PLACEMENT_3D ( 'NONE', #12857, #22356, #15325 ) ;
#30758=CYLINDRICAL_SURFACE ( 'NONE', #3606, 7.500000000000007994 ) ;
#30772=DIRECTION ( 'NONE',  ( 0.000000000000000000, 0.000000000000000000, 1.000000000000000000 ) ) ;
#30773=AXIS2_PLACEMENT_3D ( 'NONE', #2597, #11966, #21456 ) ;
#30775=DIRECTION ( 'NONE',  ( 0.000000000000000000, 0.000000000000000000, 1.000000000000000000 ) ) ;
#30778=DIRECTION ( 'NONE',  ( 1.000000000000000000, 0.000000000000000000, 0.000000000000000000 ) ) ;
#30783=AXIS2_PLACEMENT_3D ( 'NONE', #18185, #6322, #13514 ) ;
#30799=CARTESIAN_POINT ( 'NONE',  ( 0.000000000000000000, 1.699320956058915452E-16, -1.500000000000001776 ) ) ;
#30822=CIRCLE ( 'NONE', #4007, 0.7499999999999997780 ) ;
#30824=VERTEX_POINT ( 'NONE', #4186 ) ;
#30841=EDGE_LOOP ( 'NONE', ( #9440, #30117 ) ) ;
#30843=CARTESIAN_POINT ( 'NONE',  ( -8.884323311075783991, -1.438332125858144295, 21.50000000000000000 ) ) ;
#30848=DIRECTION ( 'NONE',  ( -0.000000000000000000, 1.132880637372608986E-16, -1.000000000000000000 ) ) ;
#30853=VERTEX_POINT ( 'NONE', #11985 ) ;
#30894=COLOUR_RGB('Grey',0.48,0.52,0.57);
#30895=FILL_AREA_STYLE_COLOUR('',#30894);
#30896=FILL_AREA_STYLE('',(#30895));
#30897=SURFACE_STYLE_FILL_AREA(#30896);
#30898=SURFACE_SIDE_STYLE('',(#30897));
#30899=SURFACE_STYLE_USAGE(.BOTH.,#30898);
#30900=PRESENTATION_STYLE_ASSIGNMENT((#30899));
ENDSEC;
END-ISO-10303-21;
